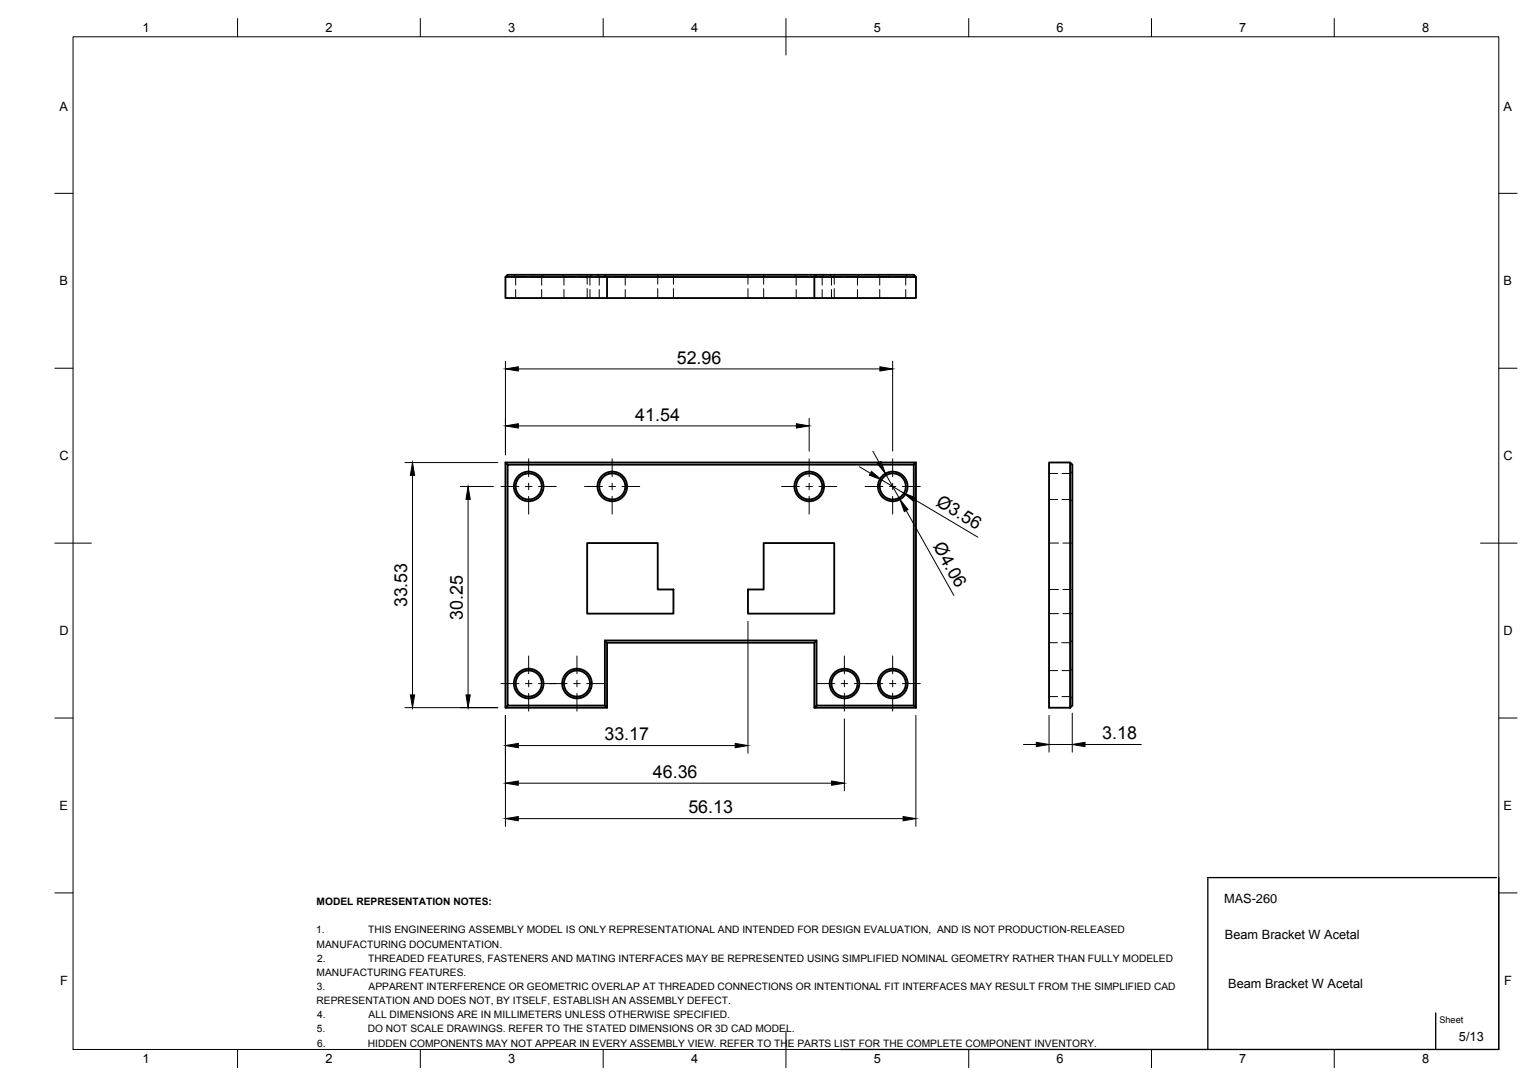
ISO-10303-21;
HEADER;
/* Generated by software containing ST-Developer
 * from STEP Tools, Inc. (www.steptools.com) 
 */

FILE_DESCRIPTION(
/* description */ (''),
/* implementation_level */ '2;1');

FILE_NAME(
/* name */ 'Beam Bracket W Acetal.step',
/* time_stamp */ '2026-10-15T13:29:10-07:00',
/* author */ (''),
/* organization */ (''),
/* preprocessor_version */ 'ST-DEVELOPER v20.2',
/* originating_system */ 'Autodesk Translation Framework v15.15.0.0',
/* authorisation */ '');

FILE_SCHEMA (('AUTOMOTIVE_DESIGN { 1 0 10303 214 3 1 1 }'));
ENDSEC;

DATA;
#10=MECHANICAL_DESIGN_GEOMETRIC_PRESENTATION_REPRESENTATION('',(#940),#83219);
#912=SHAPE_REPRESENTATION_RELATIONSHIP('SRR','None',#83307,#926);
#926=ADVANCED_BREP_SHAPE_REPRESENTATION('',(#954),#83212);
#940=STYLED_ITEM('',(#83386),#954);
#954=MANIFOLD_SOLID_BREP('Body1',#26936);
#1081=FACE_BOUND('',#4704,.T.);
#1082=FACE_BOUND('',#4705,.T.);
#1083=FACE_BOUND('',#4706,.T.);
#1084=FACE_BOUND('',#4707,.T.);
#1085=FACE_BOUND('',#4708,.T.);
#1086=FACE_BOUND('',#4709,.T.);
#1087=FACE_BOUND('',#4710,.T.);
#1088=FACE_BOUND('',#4711,.T.);
#1089=FACE_BOUND('',#4712,.T.);
#1090=FACE_BOUND('',#4713,.T.);
#1091=FACE_BOUND('',#4758,.T.);
#1092=FACE_BOUND('',#4759,.T.);
#1093=FACE_BOUND('',#4760,.T.);
#1094=FACE_BOUND('',#4761,.T.);
#1095=FACE_BOUND('',#4762,.T.);
#1096=FACE_BOUND('',#4763,.T.);
#1097=FACE_BOUND('',#4764,.T.);
#1098=FACE_BOUND('',#4765,.T.);
#1099=FACE_BOUND('',#4766,.T.);
#1100=FACE_BOUND('',#4767,.T.);
#1713=PLANE('',#28339);
#1714=PLANE('',#28377);
#1715=PLANE('',#28378);
#1716=PLANE('',#28379);
#1717=PLANE('',#28380);
#1718=PLANE('',#28381);
#1719=PLANE('',#28382);
#1720=PLANE('',#28383);
#1721=PLANE('',#28384);
#1722=PLANE('',#28385);
#1723=PLANE('',#28386);
#1724=PLANE('',#28387);
#1725=PLANE('',#28388);
#1726=PLANE('',#28389);
#1727=PLANE('',#28390);
#1728=PLANE('',#28391);
#1729=PLANE('',#28392);
#1730=PLANE('',#28393);
#1731=PLANE('',#28394);
#1732=PLANE('',#28395);
#1733=PLANE('',#28396);
#1734=PLANE('',#28397);
#1735=PLANE('',#28398);
#1736=PLANE('',#28399);
#1737=PLANE('',#28400);
#1738=PLANE('',#28401);
#1739=PLANE('',#28402);
#1740=PLANE('',#28403);
#1741=PLANE('',#28404);
#1742=PLANE('',#28405);
#2294=CYLINDRICAL_SURFACE('',#28347,1.778);
#2295=CYLINDRICAL_SURFACE('',#28351,1.778);
#2296=CYLINDRICAL_SURFACE('',#28355,1.778);
#2297=CYLINDRICAL_SURFACE('',#28359,1.778);
#2298=CYLINDRICAL_SURFACE('',#28363,1.778);
#2299=CYLINDRICAL_SURFACE('',#28367,1.778);
#2300=CYLINDRICAL_SURFACE('',#28371,1.778);
#2301=CYLINDRICAL_SURFACE('',#28375,1.778);
#3203=FACE_OUTER_BOUND('',#4702,.T.);
#3204=FACE_OUTER_BOUND('',#4703,.T.);
#3205=FACE_OUTER_BOUND('',#4714,.T.);
#3206=FACE_OUTER_BOUND('',#4715,.T.);
#3207=FACE_OUTER_BOUND('',#4716,.T.);
#3208=FACE_OUTER_BOUND('',#4717,.T.);
#3209=FACE_OUTER_BOUND('',#4718,.T.);
#3210=FACE_OUTER_BOUND('',#4719,.T.);
#3211=FACE_OUTER_BOUND('',#4720,.T.);
#3212=FACE_OUTER_BOUND('',#4721,.T.);
#3213=FACE_OUTER_BOUND('',#4722,.T.);
#3214=FACE_OUTER_BOUND('',#4723,.T.);
#3215=FACE_OUTER_BOUND('',#4724,.T.);
#3216=FACE_OUTER_BOUND('',#4725,.T.);
#3217=FACE_OUTER_BOUND('',#4726,.T.);
#3218=FACE_OUTER_BOUND('',#4727,.T.);
#3219=FACE_OUTER_BOUND('',#4728,.T.);
#3220=FACE_OUTER_BOUND('',#4729,.T.);
#3221=FACE_OUTER_BOUND('',#4730,.T.);
#3222=FACE_OUTER_BOUND('',#4731,.T.);
#3223=FACE_OUTER_BOUND('',#4732,.T.);
#3224=FACE_OUTER_BOUND('',#4733,.T.);
#3225=FACE_OUTER_BOUND('',#4734,.T.);
#3226=FACE_OUTER_BOUND('',#4735,.T.);
#3227=FACE_OUTER_BOUND('',#4736,.T.);
#3228=FACE_OUTER_BOUND('',#4737,.T.);
#3229=FACE_OUTER_BOUND('',#4738,.T.);
#3230=FACE_OUTER_BOUND('',#4739,.T.);
#3231=FACE_OUTER_BOUND('',#4740,.T.);
#3232=FACE_OUTER_BOUND('',#4741,.T.);
#3233=FACE_OUTER_BOUND('',#4742,.T.);
#3234=FACE_OUTER_BOUND('',#4743,.T.);
#3235=FACE_OUTER_BOUND('',#4744,.T.);
#3236=FACE_OUTER_BOUND('',#4745,.T.);
#3237=FACE_OUTER_BOUND('',#4746,.T.);
#3238=FACE_OUTER_BOUND('',#4747,.T.);
#3239=FACE_OUTER_BOUND('',#4748,.T.);
#3240=FACE_OUTER_BOUND('',#4749,.T.);
#3241=FACE_OUTER_BOUND('',#4750,.T.);
#3242=FACE_OUTER_BOUND('',#4751,.T.);
#3243=FACE_OUTER_BOUND('',#4752,.T.);
#3244=FACE_OUTER_BOUND('',#4753,.T.);
#3245=FACE_OUTER_BOUND('',#4754,.T.);
#3246=FACE_OUTER_BOUND('',#4755,.T.);
#3247=FACE_OUTER_BOUND('',#4756,.T.);
#3248=FACE_OUTER_BOUND('',#4757,.T.);
#4702=EDGE_LOOP('',(#22282,#22283,#22284,#22285));
#4703=EDGE_LOOP('',(#22286,#22287,#22288,#22289,#22290,#22291,#22292,#22293));
#4704=EDGE_LOOP('',(#22294));
#4705=EDGE_LOOP('',(#22295));
#4706=EDGE_LOOP('',(#22296));
#4707=EDGE_LOOP('',(#22297));
#4708=EDGE_LOOP('',(#22298,#22299,#22300,#22301,#22302,#22303));
#4709=EDGE_LOOP('',(#22304,#22305,#22306,#22307,#22308,#22309));
#4710=EDGE_LOOP('',(#22310));
#4711=EDGE_LOOP('',(#22311));
#4712=EDGE_LOOP('',(#22312));
#4713=EDGE_LOOP('',(#22313));
#4714=EDGE_LOOP('',(#22314,#22315,#22316,#22317));
#4715=EDGE_LOOP('',(#22318,#22319,#22320,#22321));
#4716=EDGE_LOOP('',(#22322,#22323,#22324,#22325));
#4717=EDGE_LOOP('',(#22326,#22327,#22328,#22329));
#4718=EDGE_LOOP('',(#22330,#22331,#22332,#22333));
#4719=EDGE_LOOP('',(#22334,#22335,#22336,#22337));
#4720=EDGE_LOOP('',(#22338,#22339,#22340,#22341));
#4721=EDGE_LOOP('',(#22342,#22343,#22344,#22345));
#4722=EDGE_LOOP('',(#22346,#22347,#22348,#22349));
#4723=EDGE_LOOP('',(#22350,#22351,#22352,#22353));
#4724=EDGE_LOOP('',(#22354,#22355,#22356,#22357));
#4725=EDGE_LOOP('',(#22358,#22359,#22360,#22361));
#4726=EDGE_LOOP('',(#22362,#22363,#22364,#22365));
#4727=EDGE_LOOP('',(#22366,#22367,#22368,#22369));
#4728=EDGE_LOOP('',(#22370,#22371,#22372,#22373));
#4729=EDGE_LOOP('',(#22374,#22375,#22376,#22377));
#4730=EDGE_LOOP('',(#22378,#22379,#22380,#22381));
#4731=EDGE_LOOP('',(#22382,#22383,#22384,#22385));
#4732=EDGE_LOOP('',(#22386,#22387,#22388,#22389));
#4733=EDGE_LOOP('',(#22390,#22391,#22392,#22393));
#4734=EDGE_LOOP('',(#22394,#22395,#22396,#22397));
#4735=EDGE_LOOP('',(#22398,#22399,#22400,#22401));
#4736=EDGE_LOOP('',(#22402,#22403,#22404,#22405));
#4737=EDGE_LOOP('',(#22406,#22407,#22408,#22409));
#4738=EDGE_LOOP('',(#22410,#22411,#22412,#22413));
#4739=EDGE_LOOP('',(#22414,#22415,#22416,#22417));
#4740=EDGE_LOOP('',(#22418,#22419,#22420,#22421));
#4741=EDGE_LOOP('',(#22422,#22423,#22424,#22425));
#4742=EDGE_LOOP('',(#22426,#22427,#22428,#22429));
#4743=EDGE_LOOP('',(#22430,#22431,#22432,#22433));
#4744=EDGE_LOOP('',(#22434,#22435,#22436,#22437));
#4745=EDGE_LOOP('',(#22438,#22439,#22440,#22441));
#4746=EDGE_LOOP('',(#22442,#22443,#22444,#22445));
#4747=EDGE_LOOP('',(#22446,#22447,#22448,#22449));
#4748=EDGE_LOOP('',(#22450,#22451,#22452,#22453));
#4749=EDGE_LOOP('',(#22454,#22455,#22456,#22457));
#4750=EDGE_LOOP('',(#22458,#22459,#22460,#22461));
#4751=EDGE_LOOP('',(#22462,#22463,#22464,#22465));
#4752=EDGE_LOOP('',(#22466,#22467,#22468,#22469));
#4753=EDGE_LOOP('',(#22470,#22471,#22472,#22473));
#4754=EDGE_LOOP('',(#22474,#22475,#22476,#22477));
#4755=EDGE_LOOP('',(#22478,#22479,#22480,#22481));
#4756=EDGE_LOOP('',(#22482,#22483,#22484,#22485));
#4757=EDGE_LOOP('',(#22486,#22487,#22488,#22489,#22490,#22491,#22492,#22493));
#4758=EDGE_LOOP('',(#22494,#22495,#22496,#22497,#22498,#22499));
#4759=EDGE_LOOP('',(#22500,#22501,#22502,#22503,#22504,#22505));
#4760=EDGE_LOOP('',(#22506));
#4761=EDGE_LOOP('',(#22507));
#4762=EDGE_LOOP('',(#22508));
#4763=EDGE_LOOP('',(#22509));
#4764=EDGE_LOOP('',(#22510));
#4765=EDGE_LOOP('',(#22511));
#4766=EDGE_LOOP('',(#22512));
#4767=EDGE_LOOP('',(#22513));
#6991=LINE('',#52756,#9502);
#6992=LINE('',#52761,#9503);
#6993=LINE('',#52763,#9504);
#6994=LINE('',#52765,#9505);
#6995=LINE('',#52767,#9506);
#6996=LINE('',#52769,#9507);
#6997=LINE('',#52771,#9508);
#6998=LINE('',#52773,#9509);
#6999=LINE('',#52774,#9510);
#7000=LINE('',#52785,#9511);
#7001=LINE('',#52787,#9512);
#7002=LINE('',#52789,#9513);
#7003=LINE('',#52791,#9514);
#7004=LINE('',#52793,#9515);
#7005=LINE('',#52794,#9516);
#7006=LINE('',#52797,#9517);
#7007=LINE('',#52799,#9518);
#7008=LINE('',#52801,#9519);
#7009=LINE('',#52803,#9520);
#7010=LINE('',#52805,#9521);
#7011=LINE('',#52806,#9522);
#7012=LINE('',#52815,#9523);
#7013=LINE('',#52820,#9524);
#7014=LINE('',#52823,#9525);
#7015=LINE('',#52828,#9526);
#7016=LINE('',#52831,#9527);
#7017=LINE('',#52836,#9528);
#7018=LINE('',#52839,#9529);
#7019=LINE('',#52844,#9530);
#7020=LINE('',#52847,#9531);
#7021=LINE('',#52852,#9532);
#7022=LINE('',#52855,#9533);
#7023=LINE('',#52860,#9534);
#7024=LINE('',#52863,#9535);
#7025=LINE('',#52868,#9536);
#7026=LINE('',#52871,#9537);
#7027=LINE('',#52876,#9538);
#7028=LINE('',#52877,#9539);
#7029=LINE('',#52878,#9540);
#7030=LINE('',#52881,#9541);
#7031=LINE('',#52882,#9542);
#7032=LINE('',#52885,#9543);
#7033=LINE('',#52886,#9544);
#7034=LINE('',#52889,#9545);
#7035=LINE('',#52890,#9546);
#7036=LINE('',#52893,#9547);
#7037=LINE('',#52894,#9548);
#7038=LINE('',#52896,#9549);
#7039=LINE('',#52900,#9550);
#7040=LINE('',#52901,#9551);
#7041=LINE('',#52902,#9552);
#7042=LINE('',#52905,#9553);
#7043=LINE('',#52906,#9554);
#7044=LINE('',#52909,#9555);
#7045=LINE('',#52910,#9556);
#7046=LINE('',#52913,#9557);
#7047=LINE('',#52914,#9558);
#7048=LINE('',#52917,#9559);
#7049=LINE('',#52918,#9560);
#7050=LINE('',#52920,#9561);
#7051=LINE('',#52923,#9562);
#7052=LINE('',#52925,#9563);
#7053=LINE('',#52926,#9564);
#7054=LINE('',#52929,#9565);
#7055=LINE('',#52930,#9566);
#7056=LINE('',#52933,#9567);
#7057=LINE('',#52934,#9568);
#7058=LINE('',#52937,#9569);
#7059=LINE('',#52938,#9570);
#7060=LINE('',#52941,#9571);
#7061=LINE('',#52942,#9572);
#7062=LINE('',#52945,#9573);
#7063=LINE('',#52946,#9574);
#7064=LINE('',#52949,#9575);
#7065=LINE('',#52950,#9576);
#7066=LINE('',#52952,#9577);
#7067=LINE('',#52955,#9578);
#7068=LINE('',#52957,#9579);
#7069=LINE('',#52958,#9580);
#7070=LINE('',#52961,#9581);
#7071=LINE('',#52962,#9582);
#7072=LINE('',#52965,#9583);
#7073=LINE('',#52966,#9584);
#7074=LINE('',#52969,#9585);
#7075=LINE('',#52970,#9586);
#7076=LINE('',#52973,#9587);
#7077=LINE('',#52974,#9588);
#7078=LINE('',#52977,#9589);
#7079=LINE('',#52978,#9590);
#7080=LINE('',#52981,#9591);
#7081=LINE('',#52982,#9592);
#7082=LINE('',#52984,#9593);
#9502=VECTOR('',#33449,1.903);
#9503=VECTOR('',#33454,10.);
#9504=VECTOR('',#33455,10.);
#9505=VECTOR('',#33456,10.);
#9506=VECTOR('',#33457,10.);
#9507=VECTOR('',#33458,10.);
#9508=VECTOR('',#33459,10.);
#9509=VECTOR('',#33460,10.);
#9510=VECTOR('',#33461,10.);
#9511=VECTOR('',#33470,10.);
#9512=VECTOR('',#33471,10.);
#9513=VECTOR('',#33472,10.);
#9514=VECTOR('',#33473,10.);
#9515=VECTOR('',#33474,10.);
#9516=VECTOR('',#33475,10.);
#9517=VECTOR('',#33476,10.);
#9518=VECTOR('',#33477,10.);
#9519=VECTOR('',#33478,10.);
#9520=VECTOR('',#33479,10.);
#9521=VECTOR('',#33480,10.);
#9522=VECTOR('',#33481,10.);
#9523=VECTOR('',#33490,1.778);
#9524=VECTOR('',#33497,1.903);
#9525=VECTOR('',#33500,1.778);
#9526=VECTOR('',#33507,1.903);
#9527=VECTOR('',#33510,1.778);
#9528=VECTOR('',#33517,1.903);
#9529=VECTOR('',#33520,1.778);
#9530=VECTOR('',#33527,1.903);
#9531=VECTOR('',#33530,1.778);
#9532=VECTOR('',#33537,1.903);
#9533=VECTOR('',#33540,1.778);
#9534=VECTOR('',#33547,1.903);
#9535=VECTOR('',#33550,1.778);
#9536=VECTOR('',#33557,1.903);
#9537=VECTOR('',#33560,1.778);
#9538=VECTOR('',#33565,10.);
#9539=VECTOR('',#33566,10.);
#9540=VECTOR('',#33567,10.);
#9541=VECTOR('',#33570,10.);
#9542=VECTOR('',#33571,10.);
#9543=VECTOR('',#33574,10.);
#9544=VECTOR('',#33575,10.);
#9545=VECTOR('',#33578,10.);
#9546=VECTOR('',#33579,10.);
#9547=VECTOR('',#33582,10.);
#9548=VECTOR('',#33583,10.);
#9549=VECTOR('',#33586,10.);
#9550=VECTOR('',#33589,10.);
#9551=VECTOR('',#33590,10.);
#9552=VECTOR('',#33591,10.);
#9553=VECTOR('',#33594,10.);
#9554=VECTOR('',#33595,10.);
#9555=VECTOR('',#33598,10.);
#9556=VECTOR('',#33599,10.);
#9557=VECTOR('',#33602,10.);
#9558=VECTOR('',#33603,10.);
#9559=VECTOR('',#33606,10.);
#9560=VECTOR('',#33607,10.);
#9561=VECTOR('',#33610,10.);
#9562=VECTOR('',#33613,10.);
#9563=VECTOR('',#33614,10.);
#9564=VECTOR('',#33615,10.);
#9565=VECTOR('',#33618,10.);
#9566=VECTOR('',#33619,10.);
#9567=VECTOR('',#33622,10.);
#9568=VECTOR('',#33623,10.);
#9569=VECTOR('',#33626,10.);
#9570=VECTOR('',#33627,10.);
#9571=VECTOR('',#33630,10.);
#9572=VECTOR('',#33631,10.);
#9573=VECTOR('',#33634,10.);
#9574=VECTOR('',#33635,10.);
#9575=VECTOR('',#33638,10.);
#9576=VECTOR('',#33639,10.);
#9577=VECTOR('',#33642,10.);
#9578=VECTOR('',#33645,10.);
#9579=VECTOR('',#33646,10.);
#9580=VECTOR('',#33647,10.);
#9581=VECTOR('',#33650,10.);
#9582=VECTOR('',#33651,10.);
#9583=VECTOR('',#33654,10.);
#9584=VECTOR('',#33655,10.);
#9585=VECTOR('',#33658,10.);
#9586=VECTOR('',#33659,10.);
#9587=VECTOR('',#33662,10.);
#9588=VECTOR('',#33663,10.);
#9589=VECTOR('',#33666,10.);
#9590=VECTOR('',#33667,10.);
#9591=VECTOR('',#33670,10.);
#9592=VECTOR('',#33671,10.);
#9593=VECTOR('',#33674,10.);
#10716=CIRCLE('',#28337,1.778);
#10717=CIRCLE('',#28338,2.028);
#10718=CIRCLE('',#28340,2.028);
#10719=CIRCLE('',#28341,2.028);
#10720=CIRCLE('',#28342,2.028);
#10721=CIRCLE('',#28343,2.028);
#10722=CIRCLE('',#28344,2.028);
#10723=CIRCLE('',#28345,2.028);
#10724=CIRCLE('',#28346,2.028);
#10725=CIRCLE('',#28348,1.778);
#10726=CIRCLE('',#28350,1.778);
#10727=CIRCLE('',#28352,1.778);
#10728=CIRCLE('',#28354,1.778);
#10729=CIRCLE('',#28356,1.778);
#10730=CIRCLE('',#28358,1.778);
#10731=CIRCLE('',#28360,1.778);
#10732=CIRCLE('',#28362,1.778);
#10733=CIRCLE('',#28364,1.778);
#10734=CIRCLE('',#28366,1.778);
#10735=CIRCLE('',#28368,1.778);
#10736=CIRCLE('',#28370,1.778);
#10737=CIRCLE('',#28372,1.778);
#10738=CIRCLE('',#28374,1.778);
#10739=CIRCLE('',#28376,1.778);
#12579=VERTEX_POINT('',#52753);
#12580=VERTEX_POINT('',#52755);
#12581=VERTEX_POINT('',#52759);
#12582=VERTEX_POINT('',#52760);
#12583=VERTEX_POINT('',#52762);
#12584=VERTEX_POINT('',#52764);
#12585=VERTEX_POINT('',#52766);
#12586=VERTEX_POINT('',#52768);
#12587=VERTEX_POINT('',#52770);
#12588=VERTEX_POINT('',#52772);
#12589=VERTEX_POINT('',#52775);
#12590=VERTEX_POINT('',#52777);
#12591=VERTEX_POINT('',#52779);
#12592=VERTEX_POINT('',#52781);
#12593=VERTEX_POINT('',#52783);
#12594=VERTEX_POINT('',#52784);
#12595=VERTEX_POINT('',#52786);
#12596=VERTEX_POINT('',#52788);
#12597=VERTEX_POINT('',#52790);
#12598=VERTEX_POINT('',#52792);
#12599=VERTEX_POINT('',#52795);
#12600=VERTEX_POINT('',#52796);
#12601=VERTEX_POINT('',#52798);
#12602=VERTEX_POINT('',#52800);
#12603=VERTEX_POINT('',#52802);
#12604=VERTEX_POINT('',#52804);
#12605=VERTEX_POINT('',#52807);
#12606=VERTEX_POINT('',#52809);
#12607=VERTEX_POINT('',#52811);
#12608=VERTEX_POINT('',#52814);
#12609=VERTEX_POINT('',#52818);
#12610=VERTEX_POINT('',#52822);
#12611=VERTEX_POINT('',#52826);
#12612=VERTEX_POINT('',#52830);
#12613=VERTEX_POINT('',#52834);
#12614=VERTEX_POINT('',#52838);
#12615=VERTEX_POINT('',#52842);
#12616=VERTEX_POINT('',#52846);
#12617=VERTEX_POINT('',#52850);
#12618=VERTEX_POINT('',#52854);
#12619=VERTEX_POINT('',#52858);
#12620=VERTEX_POINT('',#52862);
#12621=VERTEX_POINT('',#52866);
#12622=VERTEX_POINT('',#52870);
#12623=VERTEX_POINT('',#52874);
#12624=VERTEX_POINT('',#52875);
#12625=VERTEX_POINT('',#52880);
#12626=VERTEX_POINT('',#52884);
#12627=VERTEX_POINT('',#52888);
#12628=VERTEX_POINT('',#52892);
#12629=VERTEX_POINT('',#52898);
#12630=VERTEX_POINT('',#52899);
#12631=VERTEX_POINT('',#52904);
#12632=VERTEX_POINT('',#52908);
#12633=VERTEX_POINT('',#52912);
#12634=VERTEX_POINT('',#52916);
#12635=VERTEX_POINT('',#52922);
#12636=VERTEX_POINT('',#52924);
#12637=VERTEX_POINT('',#52928);
#12638=VERTEX_POINT('',#52932);
#12639=VERTEX_POINT('',#52936);
#12640=VERTEX_POINT('',#52940);
#12641=VERTEX_POINT('',#52944);
#12642=VERTEX_POINT('',#52948);
#12643=VERTEX_POINT('',#52954);
#12644=VERTEX_POINT('',#52956);
#12645=VERTEX_POINT('',#52960);
#12646=VERTEX_POINT('',#52964);
#12647=VERTEX_POINT('',#52968);
#12648=VERTEX_POINT('',#52972);
#12649=VERTEX_POINT('',#52976);
#12650=VERTEX_POINT('',#52980);
#16002=EDGE_CURVE('',#12579,#12579,#10716,.T.);
#16003=EDGE_CURVE('',#12579,#12580,#6991,.T.);
#16004=EDGE_CURVE('',#12580,#12580,#10717,.T.);
#16005=EDGE_CURVE('',#12581,#12582,#6992,.T.);
#16006=EDGE_CURVE('',#12583,#12581,#6993,.T.);
#16007=EDGE_CURVE('',#12584,#12583,#6994,.T.);
#16008=EDGE_CURVE('',#12585,#12584,#6995,.T.);
#16009=EDGE_CURVE('',#12586,#12585,#6996,.T.);
#16010=EDGE_CURVE('',#12587,#12586,#6997,.T.);
#16011=EDGE_CURVE('',#12588,#12587,#6998,.T.);
#16012=EDGE_CURVE('',#12582,#12588,#6999,.T.);
#16013=EDGE_CURVE('',#12589,#12589,#10718,.T.);
#16014=EDGE_CURVE('',#12590,#12590,#10719,.T.);
#16015=EDGE_CURVE('',#12591,#12591,#10720,.T.);
#16016=EDGE_CURVE('',#12592,#12592,#10721,.T.);
#16017=EDGE_CURVE('',#12593,#12594,#7000,.T.);
#16018=EDGE_CURVE('',#12594,#12595,#7001,.T.);
#16019=EDGE_CURVE('',#12595,#12596,#7002,.T.);
#16020=EDGE_CURVE('',#12596,#12597,#7003,.T.);
#16021=EDGE_CURVE('',#12597,#12598,#7004,.T.);
#16022=EDGE_CURVE('',#12598,#12593,#7005,.T.);
#16023=EDGE_CURVE('',#12599,#12600,#7006,.T.);
#16024=EDGE_CURVE('',#12600,#12601,#7007,.T.);
#16025=EDGE_CURVE('',#12601,#12602,#7008,.T.);
#16026=EDGE_CURVE('',#12602,#12603,#7009,.T.);
#16027=EDGE_CURVE('',#12603,#12604,#7010,.T.);
#16028=EDGE_CURVE('',#12604,#12599,#7011,.T.);
#16029=EDGE_CURVE('',#12605,#12605,#10722,.T.);
#16030=EDGE_CURVE('',#12606,#12606,#10723,.T.);
#16031=EDGE_CURVE('',#12607,#12607,#10724,.T.);
#16032=EDGE_CURVE('',#12579,#12608,#7012,.T.);
#16033=EDGE_CURVE('',#12608,#12608,#10725,.T.);
#16034=EDGE_CURVE('',#12609,#12609,#10726,.T.);
#16035=EDGE_CURVE('',#12609,#12589,#7013,.T.);
#16036=EDGE_CURVE('',#12609,#12610,#7014,.T.);
#16037=EDGE_CURVE('',#12610,#12610,#10727,.T.);
#16038=EDGE_CURVE('',#12611,#12611,#10728,.T.);
#16039=EDGE_CURVE('',#12611,#12607,#7015,.T.);
#16040=EDGE_CURVE('',#12611,#12612,#7016,.T.);
#16041=EDGE_CURVE('',#12612,#12612,#10729,.T.);
#16042=EDGE_CURVE('',#12613,#12613,#10730,.T.);
#16043=EDGE_CURVE('',#12613,#12590,#7017,.T.);
#16044=EDGE_CURVE('',#12613,#12614,#7018,.T.);
#16045=EDGE_CURVE('',#12614,#12614,#10731,.T.);
#16046=EDGE_CURVE('',#12615,#12615,#10732,.T.);
#16047=EDGE_CURVE('',#12615,#12606,#7019,.T.);
#16048=EDGE_CURVE('',#12615,#12616,#7020,.T.);
#16049=EDGE_CURVE('',#12616,#12616,#10733,.T.);
#16050=EDGE_CURVE('',#12617,#12617,#10734,.T.);
#16051=EDGE_CURVE('',#12617,#12591,#7021,.T.);
#16052=EDGE_CURVE('',#12617,#12618,#7022,.T.);
#16053=EDGE_CURVE('',#12618,#12618,#10735,.T.);
#16054=EDGE_CURVE('',#12619,#12619,#10736,.T.);
#16055=EDGE_CURVE('',#12619,#12605,#7023,.T.);
#16056=EDGE_CURVE('',#12619,#12620,#7024,.T.);
#16057=EDGE_CURVE('',#12620,#12620,#10737,.T.);
#16058=EDGE_CURVE('',#12621,#12621,#10738,.T.);
#16059=EDGE_CURVE('',#12621,#12592,#7025,.T.);
#16060=EDGE_CURVE('',#12621,#12622,#7026,.T.);
#16061=EDGE_CURVE('',#12622,#12622,#10739,.T.);
#16062=EDGE_CURVE('',#12623,#12624,#7027,.T.);
#16063=EDGE_CURVE('',#12623,#12600,#7028,.T.);
#16064=EDGE_CURVE('',#12624,#12599,#7029,.T.);
#16065=EDGE_CURVE('',#12625,#12623,#7030,.T.);
#16066=EDGE_CURVE('',#12625,#12601,#7031,.T.);
#16067=EDGE_CURVE('',#12626,#12625,#7032,.T.);
#16068=EDGE_CURVE('',#12626,#12602,#7033,.T.);
#16069=EDGE_CURVE('',#12627,#12626,#7034,.T.);
#16070=EDGE_CURVE('',#12627,#12603,#7035,.T.);
#16071=EDGE_CURVE('',#12628,#12627,#7036,.T.);
#16072=EDGE_CURVE('',#12628,#12604,#7037,.T.);
#16073=EDGE_CURVE('',#12624,#12628,#7038,.T.);
#16074=EDGE_CURVE('',#12629,#12630,#7039,.T.);
#16075=EDGE_CURVE('',#12629,#12594,#7040,.T.);
#16076=EDGE_CURVE('',#12630,#12593,#7041,.T.);
#16077=EDGE_CURVE('',#12631,#12629,#7042,.T.);
#16078=EDGE_CURVE('',#12631,#12595,#7043,.T.);
#16079=EDGE_CURVE('',#12632,#12631,#7044,.T.);
#16080=EDGE_CURVE('',#12632,#12596,#7045,.T.);
#16081=EDGE_CURVE('',#12633,#12632,#7046,.T.);
#16082=EDGE_CURVE('',#12633,#12597,#7047,.T.);
#16083=EDGE_CURVE('',#12634,#12633,#7048,.T.);
#16084=EDGE_CURVE('',#12634,#12598,#7049,.T.);
#16085=EDGE_CURVE('',#12630,#12634,#7050,.T.);
#16086=EDGE_CURVE('',#12582,#12635,#7051,.T.);
#16087=EDGE_CURVE('',#12635,#12636,#7052,.T.);
#16088=EDGE_CURVE('',#12581,#12636,#7053,.T.);
#16089=EDGE_CURVE('',#12588,#12637,#7054,.T.);
#16090=EDGE_CURVE('',#12637,#12635,#7055,.T.);
#16091=EDGE_CURVE('',#12587,#12638,#7056,.T.);
#16092=EDGE_CURVE('',#12638,#12637,#7057,.T.);
#16093=EDGE_CURVE('',#12586,#12639,#7058,.T.);
#16094=EDGE_CURVE('',#12639,#12638,#7059,.T.);
#16095=EDGE_CURVE('',#12585,#12640,#7060,.T.);
#16096=EDGE_CURVE('',#12640,#12639,#7061,.T.);
#16097=EDGE_CURVE('',#12641,#12640,#7062,.T.);
#16098=EDGE_CURVE('',#12584,#12641,#7063,.T.);
#16099=EDGE_CURVE('',#12642,#12641,#7064,.T.);
#16100=EDGE_CURVE('',#12583,#12642,#7065,.T.);
#16101=EDGE_CURVE('',#12636,#12642,#7066,.T.);
#16102=EDGE_CURVE('',#12643,#12641,#7067,.T.);
#16103=EDGE_CURVE('',#12644,#12643,#7068,.T.);
#16104=EDGE_CURVE('',#12644,#12640,#7069,.T.);
#16105=EDGE_CURVE('',#12645,#12642,#7070,.T.);
#16106=EDGE_CURVE('',#12643,#12645,#7071,.T.);
#16107=EDGE_CURVE('',#12646,#12636,#7072,.T.);
#16108=EDGE_CURVE('',#12645,#12646,#7073,.T.);
#16109=EDGE_CURVE('',#12647,#12635,#7074,.T.);
#16110=EDGE_CURVE('',#12646,#12647,#7075,.T.);
#16111=EDGE_CURVE('',#12648,#12644,#7076,.T.);
#16112=EDGE_CURVE('',#12648,#12639,#7077,.T.);
#16113=EDGE_CURVE('',#12649,#12637,#7078,.T.);
#16114=EDGE_CURVE('',#12647,#12649,#7079,.T.);
#16115=EDGE_CURVE('',#12650,#12638,#7080,.T.);
#16116=EDGE_CURVE('',#12649,#12650,#7081,.T.);
#16117=EDGE_CURVE('',#12650,#12648,#7082,.T.);
#22282=ORIENTED_EDGE('',*,*,#16002,.T.);
#22283=ORIENTED_EDGE('',*,*,#16003,.T.);
#22284=ORIENTED_EDGE('',*,*,#16004,.T.);
#22285=ORIENTED_EDGE('',*,*,#16003,.F.);
#22286=ORIENTED_EDGE('',*,*,#16005,.F.);
#22287=ORIENTED_EDGE('',*,*,#16006,.F.);
#22288=ORIENTED_EDGE('',*,*,#16007,.F.);
#22289=ORIENTED_EDGE('',*,*,#16008,.F.);
#22290=ORIENTED_EDGE('',*,*,#16009,.F.);
#22291=ORIENTED_EDGE('',*,*,#16010,.F.);
#22292=ORIENTED_EDGE('',*,*,#16011,.F.);
#22293=ORIENTED_EDGE('',*,*,#16012,.F.);
#22294=ORIENTED_EDGE('',*,*,#16013,.F.);
#22295=ORIENTED_EDGE('',*,*,#16014,.F.);
#22296=ORIENTED_EDGE('',*,*,#16015,.F.);
#22297=ORIENTED_EDGE('',*,*,#16016,.F.);
#22298=ORIENTED_EDGE('',*,*,#16017,.T.);
#22299=ORIENTED_EDGE('',*,*,#16018,.T.);
#22300=ORIENTED_EDGE('',*,*,#16019,.T.);
#22301=ORIENTED_EDGE('',*,*,#16020,.T.);
#22302=ORIENTED_EDGE('',*,*,#16021,.T.);
#22303=ORIENTED_EDGE('',*,*,#16022,.T.);
#22304=ORIENTED_EDGE('',*,*,#16023,.T.);
#22305=ORIENTED_EDGE('',*,*,#16024,.T.);
#22306=ORIENTED_EDGE('',*,*,#16025,.T.);
#22307=ORIENTED_EDGE('',*,*,#16026,.T.);
#22308=ORIENTED_EDGE('',*,*,#16027,.T.);
#22309=ORIENTED_EDGE('',*,*,#16028,.T.);
#22310=ORIENTED_EDGE('',*,*,#16029,.F.);
#22311=ORIENTED_EDGE('',*,*,#16030,.F.);
#22312=ORIENTED_EDGE('',*,*,#16031,.F.);
#22313=ORIENTED_EDGE('',*,*,#16004,.F.);
#22314=ORIENTED_EDGE('',*,*,#16002,.F.);
#22315=ORIENTED_EDGE('',*,*,#16032,.T.);
#22316=ORIENTED_EDGE('',*,*,#16033,.F.);
#22317=ORIENTED_EDGE('',*,*,#16032,.F.);
#22318=ORIENTED_EDGE('',*,*,#16034,.T.);
#22319=ORIENTED_EDGE('',*,*,#16035,.T.);
#22320=ORIENTED_EDGE('',*,*,#16013,.T.);
#22321=ORIENTED_EDGE('',*,*,#16035,.F.);
#22322=ORIENTED_EDGE('',*,*,#16034,.F.);
#22323=ORIENTED_EDGE('',*,*,#16036,.T.);
#22324=ORIENTED_EDGE('',*,*,#16037,.F.);
#22325=ORIENTED_EDGE('',*,*,#16036,.F.);
#22326=ORIENTED_EDGE('',*,*,#16038,.T.);
#22327=ORIENTED_EDGE('',*,*,#16039,.T.);
#22328=ORIENTED_EDGE('',*,*,#16031,.T.);
#22329=ORIENTED_EDGE('',*,*,#16039,.F.);
#22330=ORIENTED_EDGE('',*,*,#16038,.F.);
#22331=ORIENTED_EDGE('',*,*,#16040,.T.);
#22332=ORIENTED_EDGE('',*,*,#16041,.F.);
#22333=ORIENTED_EDGE('',*,*,#16040,.F.);
#22334=ORIENTED_EDGE('',*,*,#16042,.T.);
#22335=ORIENTED_EDGE('',*,*,#16043,.T.);
#22336=ORIENTED_EDGE('',*,*,#16014,.T.);
#22337=ORIENTED_EDGE('',*,*,#16043,.F.);
#22338=ORIENTED_EDGE('',*,*,#16042,.F.);
#22339=ORIENTED_EDGE('',*,*,#16044,.T.);
#22340=ORIENTED_EDGE('',*,*,#16045,.F.);
#22341=ORIENTED_EDGE('',*,*,#16044,.F.);
#22342=ORIENTED_EDGE('',*,*,#16046,.T.);
#22343=ORIENTED_EDGE('',*,*,#16047,.T.);
#22344=ORIENTED_EDGE('',*,*,#16030,.T.);
#22345=ORIENTED_EDGE('',*,*,#16047,.F.);
#22346=ORIENTED_EDGE('',*,*,#16046,.F.);
#22347=ORIENTED_EDGE('',*,*,#16048,.T.);
#22348=ORIENTED_EDGE('',*,*,#16049,.F.);
#22349=ORIENTED_EDGE('',*,*,#16048,.F.);
#22350=ORIENTED_EDGE('',*,*,#16050,.T.);
#22351=ORIENTED_EDGE('',*,*,#16051,.T.);
#22352=ORIENTED_EDGE('',*,*,#16015,.T.);
#22353=ORIENTED_EDGE('',*,*,#16051,.F.);
#22354=ORIENTED_EDGE('',*,*,#16050,.F.);
#22355=ORIENTED_EDGE('',*,*,#16052,.T.);
#22356=ORIENTED_EDGE('',*,*,#16053,.F.);
#22357=ORIENTED_EDGE('',*,*,#16052,.F.);
#22358=ORIENTED_EDGE('',*,*,#16054,.T.);
#22359=ORIENTED_EDGE('',*,*,#16055,.T.);
#22360=ORIENTED_EDGE('',*,*,#16029,.T.);
#22361=ORIENTED_EDGE('',*,*,#16055,.F.);
#22362=ORIENTED_EDGE('',*,*,#16054,.F.);
#22363=ORIENTED_EDGE('',*,*,#16056,.T.);
#22364=ORIENTED_EDGE('',*,*,#16057,.F.);
#22365=ORIENTED_EDGE('',*,*,#16056,.F.);
#22366=ORIENTED_EDGE('',*,*,#16058,.T.);
#22367=ORIENTED_EDGE('',*,*,#16059,.T.);
#22368=ORIENTED_EDGE('',*,*,#16016,.T.);
#22369=ORIENTED_EDGE('',*,*,#16059,.F.);
#22370=ORIENTED_EDGE('',*,*,#16058,.F.);
#22371=ORIENTED_EDGE('',*,*,#16060,.T.);
#22372=ORIENTED_EDGE('',*,*,#16061,.F.);
#22373=ORIENTED_EDGE('',*,*,#16060,.F.);
#22374=ORIENTED_EDGE('',*,*,#16062,.F.);
#22375=ORIENTED_EDGE('',*,*,#16063,.T.);
#22376=ORIENTED_EDGE('',*,*,#16023,.F.);
#22377=ORIENTED_EDGE('',*,*,#16064,.F.);
#22378=ORIENTED_EDGE('',*,*,#16065,.F.);
#22379=ORIENTED_EDGE('',*,*,#16066,.T.);
#22380=ORIENTED_EDGE('',*,*,#16024,.F.);
#22381=ORIENTED_EDGE('',*,*,#16063,.F.);
#22382=ORIENTED_EDGE('',*,*,#16067,.F.);
#22383=ORIENTED_EDGE('',*,*,#16068,.T.);
#22384=ORIENTED_EDGE('',*,*,#16025,.F.);
#22385=ORIENTED_EDGE('',*,*,#16066,.F.);
#22386=ORIENTED_EDGE('',*,*,#16069,.F.);
#22387=ORIENTED_EDGE('',*,*,#16070,.T.);
#22388=ORIENTED_EDGE('',*,*,#16026,.F.);
#22389=ORIENTED_EDGE('',*,*,#16068,.F.);
#22390=ORIENTED_EDGE('',*,*,#16071,.F.);
#22391=ORIENTED_EDGE('',*,*,#16072,.T.);
#22392=ORIENTED_EDGE('',*,*,#16027,.F.);
#22393=ORIENTED_EDGE('',*,*,#16070,.F.);
#22394=ORIENTED_EDGE('',*,*,#16073,.F.);
#22395=ORIENTED_EDGE('',*,*,#16064,.T.);
#22396=ORIENTED_EDGE('',*,*,#16028,.F.);
#22397=ORIENTED_EDGE('',*,*,#16072,.F.);
#22398=ORIENTED_EDGE('',*,*,#16074,.F.);
#22399=ORIENTED_EDGE('',*,*,#16075,.T.);
#22400=ORIENTED_EDGE('',*,*,#16017,.F.);
#22401=ORIENTED_EDGE('',*,*,#16076,.F.);
#22402=ORIENTED_EDGE('',*,*,#16077,.F.);
#22403=ORIENTED_EDGE('',*,*,#16078,.T.);
#22404=ORIENTED_EDGE('',*,*,#16018,.F.);
#22405=ORIENTED_EDGE('',*,*,#16075,.F.);
#22406=ORIENTED_EDGE('',*,*,#16079,.F.);
#22407=ORIENTED_EDGE('',*,*,#16080,.T.);
#22408=ORIENTED_EDGE('',*,*,#16019,.F.);
#22409=ORIENTED_EDGE('',*,*,#16078,.F.);
#22410=ORIENTED_EDGE('',*,*,#16081,.F.);
#22411=ORIENTED_EDGE('',*,*,#16082,.T.);
#22412=ORIENTED_EDGE('',*,*,#16020,.F.);
#22413=ORIENTED_EDGE('',*,*,#16080,.F.);
#22414=ORIENTED_EDGE('',*,*,#16083,.F.);
#22415=ORIENTED_EDGE('',*,*,#16084,.T.);
#22416=ORIENTED_EDGE('',*,*,#16021,.F.);
#22417=ORIENTED_EDGE('',*,*,#16082,.F.);
#22418=ORIENTED_EDGE('',*,*,#16085,.F.);
#22419=ORIENTED_EDGE('',*,*,#16076,.T.);
#22420=ORIENTED_EDGE('',*,*,#16022,.F.);
#22421=ORIENTED_EDGE('',*,*,#16084,.F.);
#22422=ORIENTED_EDGE('',*,*,#16005,.T.);
#22423=ORIENTED_EDGE('',*,*,#16086,.T.);
#22424=ORIENTED_EDGE('',*,*,#16087,.T.);
#22425=ORIENTED_EDGE('',*,*,#16088,.F.);
#22426=ORIENTED_EDGE('',*,*,#16012,.T.);
#22427=ORIENTED_EDGE('',*,*,#16089,.T.);
#22428=ORIENTED_EDGE('',*,*,#16090,.T.);
#22429=ORIENTED_EDGE('',*,*,#16086,.F.);
#22430=ORIENTED_EDGE('',*,*,#16011,.T.);
#22431=ORIENTED_EDGE('',*,*,#16091,.T.);
#22432=ORIENTED_EDGE('',*,*,#16092,.T.);
#22433=ORIENTED_EDGE('',*,*,#16089,.F.);
#22434=ORIENTED_EDGE('',*,*,#16010,.T.);
#22435=ORIENTED_EDGE('',*,*,#16093,.T.);
#22436=ORIENTED_EDGE('',*,*,#16094,.T.);
#22437=ORIENTED_EDGE('',*,*,#16091,.F.);
#22438=ORIENTED_EDGE('',*,*,#16009,.T.);
#22439=ORIENTED_EDGE('',*,*,#16095,.T.);
#22440=ORIENTED_EDGE('',*,*,#16096,.T.);
#22441=ORIENTED_EDGE('',*,*,#16093,.F.);
#22442=ORIENTED_EDGE('',*,*,#16097,.T.);
#22443=ORIENTED_EDGE('',*,*,#16095,.F.);
#22444=ORIENTED_EDGE('',*,*,#16008,.T.);
#22445=ORIENTED_EDGE('',*,*,#16098,.T.);
#22446=ORIENTED_EDGE('',*,*,#16099,.T.);
#22447=ORIENTED_EDGE('',*,*,#16098,.F.);
#22448=ORIENTED_EDGE('',*,*,#16007,.T.);
#22449=ORIENTED_EDGE('',*,*,#16100,.T.);
#22450=ORIENTED_EDGE('',*,*,#16101,.T.);
#22451=ORIENTED_EDGE('',*,*,#16100,.F.);
#22452=ORIENTED_EDGE('',*,*,#16006,.T.);
#22453=ORIENTED_EDGE('',*,*,#16088,.T.);
#22454=ORIENTED_EDGE('',*,*,#16097,.F.);
#22455=ORIENTED_EDGE('',*,*,#16102,.F.);
#22456=ORIENTED_EDGE('',*,*,#16103,.F.);
#22457=ORIENTED_EDGE('',*,*,#16104,.T.);
#22458=ORIENTED_EDGE('',*,*,#16099,.F.);
#22459=ORIENTED_EDGE('',*,*,#16105,.F.);
#22460=ORIENTED_EDGE('',*,*,#16106,.F.);
#22461=ORIENTED_EDGE('',*,*,#16102,.T.);
#22462=ORIENTED_EDGE('',*,*,#16101,.F.);
#22463=ORIENTED_EDGE('',*,*,#16107,.F.);
#22464=ORIENTED_EDGE('',*,*,#16108,.F.);
#22465=ORIENTED_EDGE('',*,*,#16105,.T.);
#22466=ORIENTED_EDGE('',*,*,#16087,.F.);
#22467=ORIENTED_EDGE('',*,*,#16109,.F.);
#22468=ORIENTED_EDGE('',*,*,#16110,.F.);
#22469=ORIENTED_EDGE('',*,*,#16107,.T.);
#22470=ORIENTED_EDGE('',*,*,#16096,.F.);
#22471=ORIENTED_EDGE('',*,*,#16104,.F.);
#22472=ORIENTED_EDGE('',*,*,#16111,.F.);
#22473=ORIENTED_EDGE('',*,*,#16112,.T.);
#22474=ORIENTED_EDGE('',*,*,#16090,.F.);
#22475=ORIENTED_EDGE('',*,*,#16113,.F.);
#22476=ORIENTED_EDGE('',*,*,#16114,.F.);
#22477=ORIENTED_EDGE('',*,*,#16109,.T.);
#22478=ORIENTED_EDGE('',*,*,#16092,.F.);
#22479=ORIENTED_EDGE('',*,*,#16115,.F.);
#22480=ORIENTED_EDGE('',*,*,#16116,.F.);
#22481=ORIENTED_EDGE('',*,*,#16113,.T.);
#22482=ORIENTED_EDGE('',*,*,#16094,.F.);
#22483=ORIENTED_EDGE('',*,*,#16112,.F.);
#22484=ORIENTED_EDGE('',*,*,#16117,.F.);
#22485=ORIENTED_EDGE('',*,*,#16115,.T.);
#22486=ORIENTED_EDGE('',*,*,#16117,.T.);
#22487=ORIENTED_EDGE('',*,*,#16111,.T.);
#22488=ORIENTED_EDGE('',*,*,#16103,.T.);
#22489=ORIENTED_EDGE('',*,*,#16106,.T.);
#22490=ORIENTED_EDGE('',*,*,#16108,.T.);
#22491=ORIENTED_EDGE('',*,*,#16110,.T.);
#22492=ORIENTED_EDGE('',*,*,#16114,.T.);
#22493=ORIENTED_EDGE('',*,*,#16116,.T.);
#22494=ORIENTED_EDGE('',*,*,#16074,.T.);
#22495=ORIENTED_EDGE('',*,*,#16085,.T.);
#22496=ORIENTED_EDGE('',*,*,#16083,.T.);
#22497=ORIENTED_EDGE('',*,*,#16081,.T.);
#22498=ORIENTED_EDGE('',*,*,#16079,.T.);
#22499=ORIENTED_EDGE('',*,*,#16077,.T.);
#22500=ORIENTED_EDGE('',*,*,#16062,.T.);
#22501=ORIENTED_EDGE('',*,*,#16073,.T.);
#22502=ORIENTED_EDGE('',*,*,#16071,.T.);
#22503=ORIENTED_EDGE('',*,*,#16069,.T.);
#22504=ORIENTED_EDGE('',*,*,#16067,.T.);
#22505=ORIENTED_EDGE('',*,*,#16065,.T.);
#22506=ORIENTED_EDGE('',*,*,#16033,.T.);
#22507=ORIENTED_EDGE('',*,*,#16037,.T.);
#22508=ORIENTED_EDGE('',*,*,#16041,.T.);
#22509=ORIENTED_EDGE('',*,*,#16045,.T.);
#22510=ORIENTED_EDGE('',*,*,#16049,.T.);
#22511=ORIENTED_EDGE('',*,*,#16053,.T.);
#22512=ORIENTED_EDGE('',*,*,#16057,.T.);
#22513=ORIENTED_EDGE('',*,*,#16061,.T.);
#25518=CONICAL_SURFACE('',#28336,1.903,0.785398163397448);
#25519=CONICAL_SURFACE('',#28349,1.903,0.785398163397448);
#25520=CONICAL_SURFACE('',#28353,1.903,0.785398163397448);
#25521=CONICAL_SURFACE('',#28357,1.903,0.785398163397448);
#25522=CONICAL_SURFACE('',#28361,1.903,0.785398163397448);
#25523=CONICAL_SURFACE('',#28365,1.903,0.785398163397448);
#25524=CONICAL_SURFACE('',#28369,1.903,0.785398163397448);
#25525=CONICAL_SURFACE('',#28373,1.903,0.785398163397448);
#26396=ADVANCED_FACE('',(#3203),#25518,.F.);
#26397=ADVANCED_FACE('',(#3204,#1081,#1082,#1083,#1084,#1085,#1086,#1087,
#1088,#1089,#1090),#1713,.T.);
#26398=ADVANCED_FACE('',(#3205),#2294,.F.);
#26399=ADVANCED_FACE('',(#3206),#25519,.F.);
#26400=ADVANCED_FACE('',(#3207),#2295,.F.);
#26401=ADVANCED_FACE('',(#3208),#25520,.F.);
#26402=ADVANCED_FACE('',(#3209),#2296,.F.);
#26403=ADVANCED_FACE('',(#3210),#25521,.F.);
#26404=ADVANCED_FACE('',(#3211),#2297,.F.);
#26405=ADVANCED_FACE('',(#3212),#25522,.F.);
#26406=ADVANCED_FACE('',(#3213),#2298,.F.);
#26407=ADVANCED_FACE('',(#3214),#25523,.F.);
#26408=ADVANCED_FACE('',(#3215),#2299,.F.);
#26409=ADVANCED_FACE('',(#3216),#25524,.F.);
#26410=ADVANCED_FACE('',(#3217),#2300,.F.);
#26411=ADVANCED_FACE('',(#3218),#25525,.F.);
#26412=ADVANCED_FACE('',(#3219),#2301,.F.);
#26413=ADVANCED_FACE('',(#3220),#1714,.F.);
#26414=ADVANCED_FACE('',(#3221),#1715,.F.);
#26415=ADVANCED_FACE('',(#3222),#1716,.F.);
#26416=ADVANCED_FACE('',(#3223),#1717,.F.);
#26417=ADVANCED_FACE('',(#3224),#1718,.F.);
#26418=ADVANCED_FACE('',(#3225),#1719,.F.);
#26419=ADVANCED_FACE('',(#3226),#1720,.F.);
#26420=ADVANCED_FACE('',(#3227),#1721,.F.);
#26421=ADVANCED_FACE('',(#3228),#1722,.F.);
#26422=ADVANCED_FACE('',(#3229),#1723,.F.);
#26423=ADVANCED_FACE('',(#3230),#1724,.F.);
#26424=ADVANCED_FACE('',(#3231),#1725,.F.);
#26425=ADVANCED_FACE('',(#3232),#1726,.T.);
#26426=ADVANCED_FACE('',(#3233),#1727,.T.);
#26427=ADVANCED_FACE('',(#3234),#1728,.T.);
#26428=ADVANCED_FACE('',(#3235),#1729,.T.);
#26429=ADVANCED_FACE('',(#3236),#1730,.T.);
#26430=ADVANCED_FACE('',(#3237),#1731,.T.);
#26431=ADVANCED_FACE('',(#3238),#1732,.T.);
#26432=ADVANCED_FACE('',(#3239),#1733,.T.);
#26433=ADVANCED_FACE('',(#3240),#1734,.T.);
#26434=ADVANCED_FACE('',(#3241),#1735,.T.);
#26435=ADVANCED_FACE('',(#3242),#1736,.T.);
#26436=ADVANCED_FACE('',(#3243),#1737,.T.);
#26437=ADVANCED_FACE('',(#3244),#1738,.T.);
#26438=ADVANCED_FACE('',(#3245),#1739,.T.);
#26439=ADVANCED_FACE('',(#3246),#1740,.T.);
#26440=ADVANCED_FACE('',(#3247),#1741,.T.);
#26441=ADVANCED_FACE('',(#3248,#1091,#1092,#1093,#1094,#1095,#1096,#1097,
#1098,#1099,#1100),#1742,.F.);
#26936=CLOSED_SHELL('',(#26396,#26397,#26398,#26399,#26400,#26401,#26402,
#26403,#26404,#26405,#26406,#26407,#26408,#26409,#26410,#26411,#26412,#26413,
#26414,#26415,#26416,#26417,#26418,#26419,#26420,#26421,#26422,#26423,#26424,
#26425,#26426,#26427,#26428,#26429,#26430,#26431,#26432,#26433,#26434,#26435,
#26436,#26437,#26438,#26439,#26440,#26441));
#28335=AXIS2_PLACEMENT_3D('',#52751,#33443,#33444);
#28336=AXIS2_PLACEMENT_3D('',#52752,#33445,#33446);
#28337=AXIS2_PLACEMENT_3D('',#52754,#33447,#33448);
#28338=AXIS2_PLACEMENT_3D('',#52757,#33450,#33451);
#28339=AXIS2_PLACEMENT_3D('',#52758,#33452,#33453);
#28340=AXIS2_PLACEMENT_3D('',#52776,#33462,#33463);
#28341=AXIS2_PLACEMENT_3D('',#52778,#33464,#33465);
#28342=AXIS2_PLACEMENT_3D('',#52780,#33466,#33467);
#28343=AXIS2_PLACEMENT_3D('',#52782,#33468,#33469);
#28344=AXIS2_PLACEMENT_3D('',#52808,#33482,#33483);
#28345=AXIS2_PLACEMENT_3D('',#52810,#33484,#33485);
#28346=AXIS2_PLACEMENT_3D('',#52812,#33486,#33487);
#28347=AXIS2_PLACEMENT_3D('',#52813,#33488,#33489);
#28348=AXIS2_PLACEMENT_3D('',#52816,#33491,#33492);
#28349=AXIS2_PLACEMENT_3D('',#52817,#33493,#33494);
#28350=AXIS2_PLACEMENT_3D('',#52819,#33495,#33496);
#28351=AXIS2_PLACEMENT_3D('',#52821,#33498,#33499);
#28352=AXIS2_PLACEMENT_3D('',#52824,#33501,#33502);
#28353=AXIS2_PLACEMENT_3D('',#52825,#33503,#33504);
#28354=AXIS2_PLACEMENT_3D('',#52827,#33505,#33506);
#28355=AXIS2_PLACEMENT_3D('',#52829,#33508,#33509);
#28356=AXIS2_PLACEMENT_3D('',#52832,#33511,#33512);
#28357=AXIS2_PLACEMENT_3D('',#52833,#33513,#33514);
#28358=AXIS2_PLACEMENT_3D('',#52835,#33515,#33516);
#28359=AXIS2_PLACEMENT_3D('',#52837,#33518,#33519);
#28360=AXIS2_PLACEMENT_3D('',#52840,#33521,#33522);
#28361=AXIS2_PLACEMENT_3D('',#52841,#33523,#33524);
#28362=AXIS2_PLACEMENT_3D('',#52843,#33525,#33526);
#28363=AXIS2_PLACEMENT_3D('',#52845,#33528,#33529);
#28364=AXIS2_PLACEMENT_3D('',#52848,#33531,#33532);
#28365=AXIS2_PLACEMENT_3D('',#52849,#33533,#33534);
#28366=AXIS2_PLACEMENT_3D('',#52851,#33535,#33536);
#28367=AXIS2_PLACEMENT_3D('',#52853,#33538,#33539);
#28368=AXIS2_PLACEMENT_3D('',#52856,#33541,#33542);
#28369=AXIS2_PLACEMENT_3D('',#52857,#33543,#33544);
#28370=AXIS2_PLACEMENT_3D('',#52859,#33545,#33546);
#28371=AXIS2_PLACEMENT_3D('',#52861,#33548,#33549);
#28372=AXIS2_PLACEMENT_3D('',#52864,#33551,#33552);
#28373=AXIS2_PLACEMENT_3D('',#52865,#33553,#33554);
#28374=AXIS2_PLACEMENT_3D('',#52867,#33555,#33556);
#28375=AXIS2_PLACEMENT_3D('',#52869,#33558,#33559);
#28376=AXIS2_PLACEMENT_3D('',#52872,#33561,#33562);
#28377=AXIS2_PLACEMENT_3D('',#52873,#33563,#33564);
#28378=AXIS2_PLACEMENT_3D('',#52879,#33568,#33569);
#28379=AXIS2_PLACEMENT_3D('',#52883,#33572,#33573);
#28380=AXIS2_PLACEMENT_3D('',#52887,#33576,#33577);
#28381=AXIS2_PLACEMENT_3D('',#52891,#33580,#33581);
#28382=AXIS2_PLACEMENT_3D('',#52895,#33584,#33585);
#28383=AXIS2_PLACEMENT_3D('',#52897,#33587,#33588);
#28384=AXIS2_PLACEMENT_3D('',#52903,#33592,#33593);
#28385=AXIS2_PLACEMENT_3D('',#52907,#33596,#33597);
#28386=AXIS2_PLACEMENT_3D('',#52911,#33600,#33601);
#28387=AXIS2_PLACEMENT_3D('',#52915,#33604,#33605);
#28388=AXIS2_PLACEMENT_3D('',#52919,#33608,#33609);
#28389=AXIS2_PLACEMENT_3D('',#52921,#33611,#33612);
#28390=AXIS2_PLACEMENT_3D('',#52927,#33616,#33617);
#28391=AXIS2_PLACEMENT_3D('',#52931,#33620,#33621);
#28392=AXIS2_PLACEMENT_3D('',#52935,#33624,#33625);
#28393=AXIS2_PLACEMENT_3D('',#52939,#33628,#33629);
#28394=AXIS2_PLACEMENT_3D('',#52943,#33632,#33633);
#28395=AXIS2_PLACEMENT_3D('',#52947,#33636,#33637);
#28396=AXIS2_PLACEMENT_3D('',#52951,#33640,#33641);
#28397=AXIS2_PLACEMENT_3D('',#52953,#33643,#33644);
#28398=AXIS2_PLACEMENT_3D('',#52959,#33648,#33649);
#28399=AXIS2_PLACEMENT_3D('',#52963,#33652,#33653);
#28400=AXIS2_PLACEMENT_3D('',#52967,#33656,#33657);
#28401=AXIS2_PLACEMENT_3D('',#52971,#33660,#33661);
#28402=AXIS2_PLACEMENT_3D('',#52975,#33664,#33665);
#28403=AXIS2_PLACEMENT_3D('',#52979,#33668,#33669);
#28404=AXIS2_PLACEMENT_3D('',#52983,#33672,#33673);
#28405=AXIS2_PLACEMENT_3D('',#52985,#33675,#33676);
#33443=DIRECTION('axis',(0.,0.,1.));
#33444=DIRECTION('refdir',(1.,0.,0.));
#33445=DIRECTION('center_axis',(1.,0.,0.));
#33446=DIRECTION('ref_axis',(0.,0.,-1.));
#33447=DIRECTION('center_axis',(-1.,0.,0.));
#33448=DIRECTION('ref_axis',(0.,0.,-1.));
#33449=DIRECTION('',(0.707106781186548,-8.65956056235493E-17,0.707106781186547));
#33450=DIRECTION('center_axis',(1.,0.,0.));
#33451=DIRECTION('ref_axis',(0.,0.,-1.));
#33452=DIRECTION('center_axis',(1.,0.,0.));
#33453=DIRECTION('ref_axis',(0.,0.,-1.));
#33454=DIRECTION('',(0.,-1.,0.));
#33455=DIRECTION('',(0.,0.,1.));
#33456=DIRECTION('',(0.,1.,0.));
#33457=DIRECTION('',(0.,0.,1.));
#33458=DIRECTION('',(0.,-1.,0.));
#33459=DIRECTION('',(0.,0.,-1.));
#33460=DIRECTION('',(0.,1.,0.));
#33461=DIRECTION('',(0.,0.,1.));
#33462=DIRECTION('center_axis',(1.,0.,0.));
#33463=DIRECTION('ref_axis',(0.,0.,-1.));
#33464=DIRECTION('center_axis',(1.,0.,0.));
#33465=DIRECTION('ref_axis',(0.,0.,-1.));
#33466=DIRECTION('center_axis',(1.,0.,0.));
#33467=DIRECTION('ref_axis',(0.,0.,-1.));
#33468=DIRECTION('center_axis',(1.,0.,0.));
#33469=DIRECTION('ref_axis',(0.,0.,-1.));
#33470=DIRECTION('',(0.,-1.,0.));
#33471=DIRECTION('',(0.,0.,1.));
#33472=DIRECTION('',(0.,1.,0.));
#33473=DIRECTION('',(0.,0.,-1.));
#33474=DIRECTION('',(0.,-1.,0.));
#33475=DIRECTION('',(0.,0.,-1.));
#33476=DIRECTION('',(0.,0.,-1.));
#33477=DIRECTION('',(0.,1.,0.));
#33478=DIRECTION('',(0.,0.,-1.));
#33479=DIRECTION('',(0.,-1.,0.));
#33480=DIRECTION('',(0.,0.,1.));
#33481=DIRECTION('',(0.,1.,0.));
#33482=DIRECTION('center_axis',(1.,0.,0.));
#33483=DIRECTION('ref_axis',(0.,0.,-1.));
#33484=DIRECTION('center_axis',(1.,0.,0.));
#33485=DIRECTION('ref_axis',(0.,0.,-1.));
#33486=DIRECTION('center_axis',(1.,0.,0.));
#33487=DIRECTION('ref_axis',(0.,0.,-1.));
#33488=DIRECTION('center_axis',(-1.,0.,0.));
#33489=DIRECTION('ref_axis',(0.,0.,-1.));
#33490=DIRECTION('',(-1.,0.,0.));
#33491=DIRECTION('center_axis',(1.,0.,0.));
#33492=DIRECTION('ref_axis',(0.,0.,-1.));
#33493=DIRECTION('center_axis',(1.,0.,0.));
#33494=DIRECTION('ref_axis',(0.,0.,-1.));
#33495=DIRECTION('center_axis',(-1.,0.,0.));
#33496=DIRECTION('ref_axis',(0.,0.,-1.));
#33497=DIRECTION('',(0.707106781186548,-8.65956056235493E-17,0.707106781186547));
#33498=DIRECTION('center_axis',(-1.,0.,0.));
#33499=DIRECTION('ref_axis',(0.,0.,-1.));
#33500=DIRECTION('',(-1.,0.,0.));
#33501=DIRECTION('center_axis',(1.,0.,0.));
#33502=DIRECTION('ref_axis',(0.,0.,-1.));
#33503=DIRECTION('center_axis',(1.,0.,0.));
#33504=DIRECTION('ref_axis',(0.,0.,-1.));
#33505=DIRECTION('center_axis',(-1.,0.,0.));
#33506=DIRECTION('ref_axis',(0.,0.,-1.));
#33507=DIRECTION('',(0.707106781186548,-8.65956056235493E-17,0.707106781186547));
#33508=DIRECTION('center_axis',(-1.,0.,0.));
#33509=DIRECTION('ref_axis',(0.,0.,-1.));
#33510=DIRECTION('',(-1.,0.,0.));
#33511=DIRECTION('center_axis',(1.,0.,0.));
#33512=DIRECTION('ref_axis',(0.,0.,-1.));
#33513=DIRECTION('center_axis',(1.,0.,0.));
#33514=DIRECTION('ref_axis',(0.,0.,-1.));
#33515=DIRECTION('center_axis',(-1.,0.,0.));
#33516=DIRECTION('ref_axis',(0.,0.,-1.));
#33517=DIRECTION('',(0.707106781186548,-8.65956056235493E-17,0.707106781186547));
#33518=DIRECTION('center_axis',(-1.,0.,0.));
#33519=DIRECTION('ref_axis',(0.,0.,-1.));
#33520=DIRECTION('',(-1.,0.,0.));
#33521=DIRECTION('center_axis',(1.,0.,0.));
#33522=DIRECTION('ref_axis',(0.,0.,-1.));
#33523=DIRECTION('center_axis',(1.,0.,0.));
#33524=DIRECTION('ref_axis',(0.,0.,-1.));
#33525=DIRECTION('center_axis',(-1.,0.,0.));
#33526=DIRECTION('ref_axis',(0.,0.,-1.));
#33527=DIRECTION('',(0.707106781186548,-8.65956056235493E-17,0.707106781186547));
#33528=DIRECTION('center_axis',(-1.,0.,0.));
#33529=DIRECTION('ref_axis',(0.,0.,-1.));
#33530=DIRECTION('',(-1.,0.,0.));
#33531=DIRECTION('center_axis',(1.,0.,0.));
#33532=DIRECTION('ref_axis',(0.,0.,-1.));
#33533=DIRECTION('center_axis',(1.,0.,0.));
#33534=DIRECTION('ref_axis',(0.,0.,-1.));
#33535=DIRECTION('center_axis',(-1.,0.,0.));
#33536=DIRECTION('ref_axis',(0.,0.,-1.));
#33537=DIRECTION('',(0.707106781186548,-8.65956056235493E-17,0.707106781186547));
#33538=DIRECTION('center_axis',(-1.,0.,0.));
#33539=DIRECTION('ref_axis',(0.,0.,-1.));
#33540=DIRECTION('',(-1.,0.,0.));
#33541=DIRECTION('center_axis',(1.,0.,0.));
#33542=DIRECTION('ref_axis',(0.,0.,-1.));
#33543=DIRECTION('center_axis',(1.,0.,0.));
#33544=DIRECTION('ref_axis',(0.,0.,-1.));
#33545=DIRECTION('center_axis',(-1.,0.,0.));
#33546=DIRECTION('ref_axis',(0.,0.,-1.));
#33547=DIRECTION('',(0.707106781186548,-8.65956056235493E-17,0.707106781186547));
#33548=DIRECTION('center_axis',(-1.,0.,0.));
#33549=DIRECTION('ref_axis',(0.,0.,-1.));
#33550=DIRECTION('',(-1.,0.,0.));
#33551=DIRECTION('center_axis',(1.,0.,0.));
#33552=DIRECTION('ref_axis',(0.,0.,-1.));
#33553=DIRECTION('center_axis',(1.,0.,0.));
#33554=DIRECTION('ref_axis',(0.,0.,-1.));
#33555=DIRECTION('center_axis',(-1.,0.,0.));
#33556=DIRECTION('ref_axis',(0.,0.,-1.));
#33557=DIRECTION('',(0.707106781186548,-8.65956056235493E-17,0.707106781186547));
#33558=DIRECTION('center_axis',(-1.,0.,0.));
#33559=DIRECTION('ref_axis',(0.,0.,-1.));
#33560=DIRECTION('',(-1.,0.,0.));
#33561=DIRECTION('center_axis',(1.,0.,0.));
#33562=DIRECTION('ref_axis',(0.,0.,-1.));
#33563=DIRECTION('center_axis',(0.,1.,0.));
#33564=DIRECTION('ref_axis',(0.,0.,1.));
#33565=DIRECTION('',(0.,0.,1.));
#33566=DIRECTION('',(1.,0.,0.));
#33567=DIRECTION('',(1.,0.,0.));
#33568=DIRECTION('center_axis',(0.,0.,1.));
#33569=DIRECTION('ref_axis',(0.,-1.,0.));
#33570=DIRECTION('',(0.,-1.,0.));
#33571=DIRECTION('',(1.,0.,0.));
#33572=DIRECTION('center_axis',(0.,1.,0.));
#33573=DIRECTION('ref_axis',(0.,0.,1.));
#33574=DIRECTION('',(0.,0.,1.));
#33575=DIRECTION('',(1.,0.,0.));
#33576=DIRECTION('center_axis',(0.,0.,-1.));
#33577=DIRECTION('ref_axis',(0.,1.,0.));
#33578=DIRECTION('',(0.,1.,0.));
#33579=DIRECTION('',(1.,0.,0.));
#33580=DIRECTION('center_axis',(0.,-1.,0.));
#33581=DIRECTION('ref_axis',(0.,0.,-1.));
#33582=DIRECTION('',(0.,0.,-1.));
#33583=DIRECTION('',(1.,0.,0.));
#33584=DIRECTION('center_axis',(0.,0.,1.));
#33585=DIRECTION('ref_axis',(0.,-1.,0.));
#33586=DIRECTION('',(0.,-1.,0.));
#33587=DIRECTION('center_axis',(0.,0.,-1.));
#33588=DIRECTION('ref_axis',(0.,1.,0.));
#33589=DIRECTION('',(0.,1.,0.));
#33590=DIRECTION('',(1.,0.,0.));
#33591=DIRECTION('',(1.,0.,0.));
#33592=DIRECTION('center_axis',(0.,-1.,0.));
#33593=DIRECTION('ref_axis',(0.,0.,-1.));
#33594=DIRECTION('',(0.,0.,-1.));
#33595=DIRECTION('',(1.,0.,0.));
#33596=DIRECTION('center_axis',(0.,0.,1.));
#33597=DIRECTION('ref_axis',(0.,-1.,0.));
#33598=DIRECTION('',(0.,-1.,0.));
#33599=DIRECTION('',(1.,0.,0.));
#33600=DIRECTION('center_axis',(0.,1.,0.));
#33601=DIRECTION('ref_axis',(0.,0.,1.));
#33602=DIRECTION('',(0.,0.,1.));
#33603=DIRECTION('',(1.,0.,0.));
#33604=DIRECTION('center_axis',(0.,0.,-1.));
#33605=DIRECTION('ref_axis',(0.,1.,0.));
#33606=DIRECTION('',(0.,1.,0.));
#33607=DIRECTION('',(1.,0.,0.));
#33608=DIRECTION('center_axis',(0.,1.,0.));
#33609=DIRECTION('ref_axis',(0.,0.,1.));
#33610=DIRECTION('',(0.,0.,1.));
#33611=DIRECTION('center_axis',(0.707106781186545,0.,-0.70710678118655));
#33612=DIRECTION('ref_axis',(-0.70710678118655,0.,-0.707106781186545));
#33613=DIRECTION('',(-0.577350269189627,-0.577350269189627,-0.577350269189623));
#33614=DIRECTION('',(0.,1.,0.));
#33615=DIRECTION('',(-0.577350269189627,-0.577350269189627,-0.577350269189623));
#33616=DIRECTION('center_axis',(0.707106781186548,-0.707106781186548,0.));
#33617=DIRECTION('ref_axis',(0.,0.,-1.));
#33618=DIRECTION('',(-0.577350269189629,-0.577350269189629,0.57735026918962));
#33619=DIRECTION('',(0.,0.,-1.));
#33620=DIRECTION('center_axis',(0.707106781186542,0.,0.707106781186553));
#33621=DIRECTION('ref_axis',(0.707106781186553,0.,-0.707106781186542));
#33622=DIRECTION('',(-0.577350269189629,0.577350269189629,0.57735026918962));
#33623=DIRECTION('',(0.,-1.,0.));
#33624=DIRECTION('center_axis',(0.707106781186548,0.707106781186548,0.));
#33625=DIRECTION('ref_axis',(0.,0.,-1.));
#33626=DIRECTION('',(-0.577350269189629,0.577350269189629,-0.57735026918962));
#33627=DIRECTION('',(0.,0.,1.));
#33628=DIRECTION('center_axis',(0.707106781186542,0.,-0.707106781186553));
#33629=DIRECTION('ref_axis',(-0.707106781186553,0.,-0.707106781186542));
#33630=DIRECTION('',(-0.577350269189629,-0.577350269189629,-0.57735026918962));
#33631=DIRECTION('',(0.,1.,0.));
#33632=DIRECTION('center_axis',(0.707106781186548,-0.707106781186548,0.));
#33633=DIRECTION('ref_axis',(0.,0.,-1.));
#33634=DIRECTION('',(0.,0.,-1.));
#33635=DIRECTION('',(-0.577350269189627,-0.577350269189627,0.577350269189623));
#33636=DIRECTION('center_axis',(0.707106781186545,0.,0.70710678118655));
#33637=DIRECTION('ref_axis',(0.70710678118655,0.,-0.707106781186545));
#33638=DIRECTION('',(0.,-1.,0.));
#33639=DIRECTION('',(-0.577350269189626,-0.577350269189626,0.577350269189626));
#33640=DIRECTION('center_axis',(0.707106781186548,-0.707106781186548,0.));
#33641=DIRECTION('ref_axis',(0.,0.,-1.));
#33642=DIRECTION('',(0.,0.,-1.));
#33643=DIRECTION('center_axis',(0.,-1.,0.));
#33644=DIRECTION('ref_axis',(0.,0.,-1.));
#33645=DIRECTION('',(1.,0.,0.));
#33646=DIRECTION('',(0.,0.,1.));
#33647=DIRECTION('',(1.,0.,0.));
#33648=DIRECTION('center_axis',(0.,0.,1.));
#33649=DIRECTION('ref_axis',(0.,-1.,0.));
#33650=DIRECTION('',(1.,0.,0.));
#33651=DIRECTION('',(0.,1.,0.));
#33652=DIRECTION('center_axis',(0.,-1.,0.));
#33653=DIRECTION('ref_axis',(0.,0.,-1.));
#33654=DIRECTION('',(1.,0.,0.));
#33655=DIRECTION('',(0.,0.,1.));
#33656=DIRECTION('center_axis',(0.,0.,-1.));
#33657=DIRECTION('ref_axis',(0.,1.,0.));
#33658=DIRECTION('',(1.,0.,0.));
#33659=DIRECTION('',(0.,-1.,0.));
#33660=DIRECTION('center_axis',(0.,0.,-1.));
#33661=DIRECTION('ref_axis',(0.,1.,0.));
#33662=DIRECTION('',(0.,-1.,0.));
#33663=DIRECTION('',(1.,0.,0.));
#33664=DIRECTION('center_axis',(0.,-1.,0.));
#33665=DIRECTION('ref_axis',(0.,0.,-1.));
#33666=DIRECTION('',(1.,0.,0.));
#33667=DIRECTION('',(0.,0.,1.));
#33668=DIRECTION('center_axis',(0.,0.,1.));
#33669=DIRECTION('ref_axis',(0.,-1.,0.));
#33670=DIRECTION('',(1.,0.,0.));
#33671=DIRECTION('',(0.,1.,0.));
#33672=DIRECTION('center_axis',(0.,1.,0.));
#33673=DIRECTION('ref_axis',(0.,0.,1.));
#33674=DIRECTION('',(0.,0.,-1.));
#33675=DIRECTION('center_axis',(1.,0.,0.));
#33676=DIRECTION('ref_axis',(0.,0.,-1.));
#52751=CARTESIAN_POINT('',(0.,0.,0.));
#52752=CARTESIAN_POINT('Origin',(19.814,44.696,24.89));
#52753=CARTESIAN_POINT('',(19.689,44.696,26.668));
#52754=CARTESIAN_POINT('Origin',(19.689,44.696,24.89));
#52755=CARTESIAN_POINT('',(19.939,44.696,26.918));
#52756=CARTESIAN_POINT('',(19.814,44.696,26.793));
#52757=CARTESIAN_POINT('Origin',(19.939,44.696,24.89));
#52758=CARTESIAN_POINT('Origin',(19.939,58.158,0.));
#52759=CARTESIAN_POINT('',(19.939,50.584,14.4732));
#52760=CARTESIAN_POINT('',(19.939,41.694,14.4732));
#52761=CARTESIAN_POINT('',(19.939,49.776,14.4732));
#52762=CARTESIAN_POINT('',(19.939,50.584,-14.4732));
#52763=CARTESIAN_POINT('',(19.939,50.584,7.0866));
#52764=CARTESIAN_POINT('',(19.939,41.694,-14.4732));
#52765=CARTESIAN_POINT('',(19.939,54.221,-14.4732));
#52766=CARTESIAN_POINT('',(19.939,41.694,-27.767));
#52767=CARTESIAN_POINT('',(19.939,41.694,-7.0866));
#52768=CARTESIAN_POINT('',(19.939,74.622,-27.767));
#52769=CARTESIAN_POINT('',(19.939,49.776,-27.767));
#52770=CARTESIAN_POINT('',(19.939,74.622,27.767));
#52771=CARTESIAN_POINT('',(19.939,74.622,-14.0335));
#52772=CARTESIAN_POINT('',(19.939,41.694,27.767));
#52773=CARTESIAN_POINT('',(19.939,66.54,27.767));
#52774=CARTESIAN_POINT('',(19.939,41.694,14.0335));
#52775=CARTESIAN_POINT('',(19.939,44.696,-16.262));
#52776=CARTESIAN_POINT('Origin',(19.939,44.696,-18.29));
#52777=CARTESIAN_POINT('',(19.939,71.6454,15.498));
#52778=CARTESIAN_POINT('Origin',(19.939,71.6454,13.47));
#52779=CARTESIAN_POINT('',(19.939,71.6454,26.918));
#52780=CARTESIAN_POINT('Origin',(19.939,71.6454,24.89));
#52781=CARTESIAN_POINT('',(19.939,44.696,20.318));
#52782=CARTESIAN_POINT('Origin',(19.939,44.696,18.29));
#52783=CARTESIAN_POINT('',(19.939,57.565,5.1));
#52784=CARTESIAN_POINT('',(19.939,54.26,5.1));
#52785=CARTESIAN_POINT('',(19.939,56.209,5.1));
#52786=CARTESIAN_POINT('',(19.939,54.26,16.892));
#52787=CARTESIAN_POINT('',(19.939,54.26,8.446));
#52788=CARTESIAN_POINT('',(19.939,63.912,16.892));
#52789=CARTESIAN_POINT('',(19.939,61.035,16.892));
#52790=CARTESIAN_POINT('',(19.939,63.912,7.24));
#52791=CARTESIAN_POINT('',(19.939,63.912,3.62));
#52792=CARTESIAN_POINT('',(19.939,57.565,7.24));
#52793=CARTESIAN_POINT('',(19.939,57.8615,7.24));
#52794=CARTESIAN_POINT('',(19.939,57.565,2.55));
#52795=CARTESIAN_POINT('',(19.939,57.565,-5.1));
#52796=CARTESIAN_POINT('',(19.939,57.565,-7.24));
#52797=CARTESIAN_POINT('',(19.939,57.565,-3.62));
#52798=CARTESIAN_POINT('',(19.939,63.912,-7.24));
#52799=CARTESIAN_POINT('',(19.939,61.035,-7.24));
#52800=CARTESIAN_POINT('',(19.939,63.912,-16.892));
#52801=CARTESIAN_POINT('',(19.939,63.912,-8.446));
#52802=CARTESIAN_POINT('',(19.939,54.26,-16.892));
#52803=CARTESIAN_POINT('',(19.939,56.209,-16.892));
#52804=CARTESIAN_POINT('',(19.939,54.26,-5.1));
#52805=CARTESIAN_POINT('',(19.939,54.26,-2.55));
#52806=CARTESIAN_POINT('',(19.939,57.8615,-5.1));
#52807=CARTESIAN_POINT('',(19.939,44.696,-22.862));
#52808=CARTESIAN_POINT('Origin',(19.939,44.696,-24.89));
#52809=CARTESIAN_POINT('',(19.939,71.6454,-11.442));
#52810=CARTESIAN_POINT('Origin',(19.939,71.6454,-13.47));
#52811=CARTESIAN_POINT('',(19.939,71.6454,-22.862));
#52812=CARTESIAN_POINT('Origin',(19.939,71.6454,-24.89));
#52813=CARTESIAN_POINT('Origin',(19.939,44.696,24.89));
#52814=CARTESIAN_POINT('',(16.764,44.696,26.668));
#52815=CARTESIAN_POINT('',(19.939,44.696,26.668));
#52816=CARTESIAN_POINT('Origin',(16.764,44.696,24.89));
#52817=CARTESIAN_POINT('Origin',(19.814,44.696,-18.29));
#52818=CARTESIAN_POINT('',(19.689,44.696,-16.512));
#52819=CARTESIAN_POINT('Origin',(19.689,44.696,-18.29));
#52820=CARTESIAN_POINT('',(19.814,44.696,-16.387));
#52821=CARTESIAN_POINT('Origin',(19.939,44.696,-18.29));
#52822=CARTESIAN_POINT('',(16.764,44.696,-16.512));
#52823=CARTESIAN_POINT('',(19.939,44.696,-16.512));
#52824=CARTESIAN_POINT('Origin',(16.764,44.696,-18.29));
#52825=CARTESIAN_POINT('Origin',(19.814,71.6454,-24.89));
#52826=CARTESIAN_POINT('',(19.689,71.6454,-23.112));
#52827=CARTESIAN_POINT('Origin',(19.689,71.6454,-24.89));
#52828=CARTESIAN_POINT('',(19.814,71.6454,-22.987));
#52829=CARTESIAN_POINT('Origin',(19.939,71.6454,-24.89));
#52830=CARTESIAN_POINT('',(16.764,71.6454,-23.112));
#52831=CARTESIAN_POINT('',(19.939,71.6454,-23.112));
#52832=CARTESIAN_POINT('Origin',(16.764,71.6454,-24.89));
#52833=CARTESIAN_POINT('Origin',(19.814,71.6454,13.47));
#52834=CARTESIAN_POINT('',(19.689,71.6454,15.248));
#52835=CARTESIAN_POINT('Origin',(19.689,71.6454,13.47));
#52836=CARTESIAN_POINT('',(19.814,71.6454,15.373));
#52837=CARTESIAN_POINT('Origin',(19.939,71.6454,13.47));
#52838=CARTESIAN_POINT('',(16.764,71.6454,15.248));
#52839=CARTESIAN_POINT('',(19.939,71.6454,15.248));
#52840=CARTESIAN_POINT('Origin',(16.764,71.6454,13.47));
#52841=CARTESIAN_POINT('Origin',(19.814,71.6454,-13.47));
#52842=CARTESIAN_POINT('',(19.689,71.6454,-11.692));
#52843=CARTESIAN_POINT('Origin',(19.689,71.6454,-13.47));
#52844=CARTESIAN_POINT('',(19.814,71.6454,-11.567));
#52845=CARTESIAN_POINT('Origin',(19.939,71.6454,-13.47));
#52846=CARTESIAN_POINT('',(16.764,71.6454,-11.692));
#52847=CARTESIAN_POINT('',(19.939,71.6454,-11.692));
#52848=CARTESIAN_POINT('Origin',(16.764,71.6454,-13.47));
#52849=CARTESIAN_POINT('Origin',(19.814,71.6454,24.89));
#52850=CARTESIAN_POINT('',(19.689,71.6454,26.668));
#52851=CARTESIAN_POINT('Origin',(19.689,71.6454,24.89));
#52852=CARTESIAN_POINT('',(19.814,71.6454,26.793));
#52853=CARTESIAN_POINT('Origin',(19.939,71.6454,24.89));
#52854=CARTESIAN_POINT('',(16.764,71.6454,26.668));
#52855=CARTESIAN_POINT('',(19.939,71.6454,26.668));
#52856=CARTESIAN_POINT('Origin',(16.764,71.6454,24.89));
#52857=CARTESIAN_POINT('Origin',(19.814,44.696,-24.89));
#52858=CARTESIAN_POINT('',(19.689,44.696,-23.112));
#52859=CARTESIAN_POINT('Origin',(19.689,44.696,-24.89));
#52860=CARTESIAN_POINT('',(19.814,44.696,-22.987));
#52861=CARTESIAN_POINT('Origin',(19.939,44.696,-24.89));
#52862=CARTESIAN_POINT('',(16.764,44.696,-23.112));
#52863=CARTESIAN_POINT('',(19.939,44.696,-23.112));
#52864=CARTESIAN_POINT('Origin',(16.764,44.696,-24.89));
#52865=CARTESIAN_POINT('Origin',(19.814,44.696,18.29));
#52866=CARTESIAN_POINT('',(19.689,44.696,20.068));
#52867=CARTESIAN_POINT('Origin',(19.689,44.696,18.29));
#52868=CARTESIAN_POINT('',(19.814,44.696,20.193));
#52869=CARTESIAN_POINT('Origin',(19.939,44.696,18.29));
#52870=CARTESIAN_POINT('',(16.764,44.696,20.068));
#52871=CARTESIAN_POINT('',(19.939,44.696,20.068));
#52872=CARTESIAN_POINT('Origin',(16.764,44.696,18.29));
#52873=CARTESIAN_POINT('Origin',(16.764,57.565,-7.24));
#52874=CARTESIAN_POINT('',(16.764,57.565,-7.24));
#52875=CARTESIAN_POINT('',(16.764,57.565,-5.1));
#52876=CARTESIAN_POINT('',(16.764,57.565,-3.62));
#52877=CARTESIAN_POINT('',(16.764,57.565,-7.24));
#52878=CARTESIAN_POINT('',(16.764,57.565,-5.1));
#52879=CARTESIAN_POINT('Origin',(16.764,63.912,-7.24));
#52880=CARTESIAN_POINT('',(16.764,63.912,-7.24));
#52881=CARTESIAN_POINT('',(16.764,61.035,-7.24));
#52882=CARTESIAN_POINT('',(16.764,63.912,-7.24));
#52883=CARTESIAN_POINT('Origin',(16.764,63.912,-16.892));
#52884=CARTESIAN_POINT('',(16.764,63.912,-16.892));
#52885=CARTESIAN_POINT('',(16.764,63.912,-8.446));
#52886=CARTESIAN_POINT('',(16.764,63.912,-16.892));
#52887=CARTESIAN_POINT('Origin',(16.764,54.26,-16.892));
#52888=CARTESIAN_POINT('',(16.764,54.26,-16.892));
#52889=CARTESIAN_POINT('',(16.764,56.209,-16.892));
#52890=CARTESIAN_POINT('',(16.764,54.26,-16.892));
#52891=CARTESIAN_POINT('Origin',(16.764,54.26,-5.1));
#52892=CARTESIAN_POINT('',(16.764,54.26,-5.1));
#52893=CARTESIAN_POINT('',(16.764,54.26,-2.55));
#52894=CARTESIAN_POINT('',(16.764,54.26,-5.1));
#52895=CARTESIAN_POINT('Origin',(16.764,57.565,-5.1));
#52896=CARTESIAN_POINT('',(16.764,57.8615,-5.1));
#52897=CARTESIAN_POINT('Origin',(16.764,54.26,5.1));
#52898=CARTESIAN_POINT('',(16.764,54.26,5.1));
#52899=CARTESIAN_POINT('',(16.764,57.565,5.1));
#52900=CARTESIAN_POINT('',(16.764,56.209,5.1));
#52901=CARTESIAN_POINT('',(16.764,54.26,5.1));
#52902=CARTESIAN_POINT('',(16.764,57.565,5.1));
#52903=CARTESIAN_POINT('Origin',(16.764,54.26,16.892));
#52904=CARTESIAN_POINT('',(16.764,54.26,16.892));
#52905=CARTESIAN_POINT('',(16.764,54.26,8.446));
#52906=CARTESIAN_POINT('',(16.764,54.26,16.892));
#52907=CARTESIAN_POINT('Origin',(16.764,63.912,16.892));
#52908=CARTESIAN_POINT('',(16.764,63.912,16.892));
#52909=CARTESIAN_POINT('',(16.764,61.035,16.892));
#52910=CARTESIAN_POINT('',(16.764,63.912,16.892));
#52911=CARTESIAN_POINT('Origin',(16.764,63.912,7.24));
#52912=CARTESIAN_POINT('',(16.764,63.912,7.24));
#52913=CARTESIAN_POINT('',(16.764,63.912,3.62));
#52914=CARTESIAN_POINT('',(16.764,63.912,7.24));
#52915=CARTESIAN_POINT('Origin',(16.764,57.565,7.24));
#52916=CARTESIAN_POINT('',(16.764,57.565,7.24));
#52917=CARTESIAN_POINT('',(16.764,57.8615,7.24));
#52918=CARTESIAN_POINT('',(16.764,57.565,7.24));
#52919=CARTESIAN_POINT('Origin',(16.764,57.565,5.1));
#52920=CARTESIAN_POINT('',(16.764,57.565,2.55));
#52921=CARTESIAN_POINT('Origin',(19.789,49.776,14.3232));
#52922=CARTESIAN_POINT('',(19.639,41.394,14.1732));
#52923=CARTESIAN_POINT('',(19.939,41.694,14.4732));
#52924=CARTESIAN_POINT('',(19.639,50.284,14.1732));
#52925=CARTESIAN_POINT('',(19.639,49.776,14.1732));
#52926=CARTESIAN_POINT('',(19.939,50.584,14.4732));
#52927=CARTESIAN_POINT('Origin',(19.789,41.544,14.0335));
#52928=CARTESIAN_POINT('',(19.639,41.394,28.067));
#52929=CARTESIAN_POINT('',(19.939,41.694,27.767));
#52930=CARTESIAN_POINT('',(19.639,41.394,14.0335));
#52931=CARTESIAN_POINT('Origin',(19.789,66.54,27.917));
#52932=CARTESIAN_POINT('',(19.639,74.922,28.067));
#52933=CARTESIAN_POINT('',(19.939,74.622,27.767));
#52934=CARTESIAN_POINT('',(19.639,66.54,28.067));
#52935=CARTESIAN_POINT('Origin',(19.789,74.772,-14.0335));
#52936=CARTESIAN_POINT('',(19.639,74.922,-28.067));
#52937=CARTESIAN_POINT('',(19.939,74.622,-27.767));
#52938=CARTESIAN_POINT('',(19.639,74.922,-14.0335));
#52939=CARTESIAN_POINT('Origin',(19.789,49.776,-27.917));
#52940=CARTESIAN_POINT('',(19.639,41.394,-28.067));
#52941=CARTESIAN_POINT('',(19.939,41.694,-27.767));
#52942=CARTESIAN_POINT('',(19.639,49.776,-28.067));
#52943=CARTESIAN_POINT('Origin',(19.789,41.544,-7.0866));
#52944=CARTESIAN_POINT('',(19.639,41.394,-14.1732));
#52945=CARTESIAN_POINT('',(19.639,41.394,-7.0866));
#52946=CARTESIAN_POINT('',(19.939,41.694,-14.4732));
#52947=CARTESIAN_POINT('Origin',(19.789,54.221,-14.3232));
#52948=CARTESIAN_POINT('',(19.639,50.284,-14.1732));
#52949=CARTESIAN_POINT('',(19.639,54.221,-14.1732));
#52950=CARTESIAN_POINT('',(19.939,50.584,-14.4732));
#52951=CARTESIAN_POINT('Origin',(19.789,50.434,7.0866));
#52952=CARTESIAN_POINT('',(19.639,50.284,7.0866));
#52953=CARTESIAN_POINT('Origin',(16.764,41.394,-14.1732));
#52954=CARTESIAN_POINT('',(16.764,41.394,-14.1732));
#52955=CARTESIAN_POINT('',(16.764,41.394,-14.1732));
#52956=CARTESIAN_POINT('',(16.764,41.394,-28.067));
#52957=CARTESIAN_POINT('',(16.764,41.394,-28.067));
#52958=CARTESIAN_POINT('',(16.764,41.394,-28.067));
#52959=CARTESIAN_POINT('Origin',(16.764,50.284,-14.1732));
#52960=CARTESIAN_POINT('',(16.764,50.284,-14.1732));
#52961=CARTESIAN_POINT('',(16.764,50.284,-14.1732));
#52962=CARTESIAN_POINT('',(16.764,41.394,-14.1732));
#52963=CARTESIAN_POINT('Origin',(16.764,50.284,14.1732));
#52964=CARTESIAN_POINT('',(16.764,50.284,14.1732));
#52965=CARTESIAN_POINT('',(16.764,50.284,14.1732));
#52966=CARTESIAN_POINT('',(16.764,50.284,-14.1732));
#52967=CARTESIAN_POINT('Origin',(16.764,41.394,14.1732));
#52968=CARTESIAN_POINT('',(16.764,41.394,14.1732));
#52969=CARTESIAN_POINT('',(16.764,41.394,14.1732));
#52970=CARTESIAN_POINT('',(16.764,50.284,14.1732));
#52971=CARTESIAN_POINT('Origin',(16.764,41.394,-28.067));
#52972=CARTESIAN_POINT('',(16.764,74.922,-28.067));
#52973=CARTESIAN_POINT('',(16.764,74.922,-28.067));
#52974=CARTESIAN_POINT('',(16.764,74.922,-28.067));
#52975=CARTESIAN_POINT('Origin',(16.764,41.394,28.067));
#52976=CARTESIAN_POINT('',(16.764,41.394,28.067));
#52977=CARTESIAN_POINT('',(16.764,41.394,28.067));
#52978=CARTESIAN_POINT('',(16.764,41.394,14.1732));
#52979=CARTESIAN_POINT('Origin',(16.764,74.922,28.067));
#52980=CARTESIAN_POINT('',(16.764,74.922,28.067));
#52981=CARTESIAN_POINT('',(16.764,74.922,28.067));
#52982=CARTESIAN_POINT('',(16.764,41.394,28.067));
#52983=CARTESIAN_POINT('Origin',(16.764,74.922,-28.067));
#52984=CARTESIAN_POINT('',(16.764,74.922,28.067));
#52985=CARTESIAN_POINT('Origin',(16.764,58.158,0.));
#83196=UNCERTAINTY_MEASURE_WITH_UNIT(LENGTH_MEASURE(0.01),#83220,
'DISTANCE_ACCURACY_VALUE',
'Maximum model space distance between geometric entities at asserted c
onnectivities');
#83203=UNCERTAINTY_MEASURE_WITH_UNIT(LENGTH_MEASURE(0.01),#83220,
'DISTANCE_ACCURACY_VALUE',
'Maximum model space distance between geometric entities at asserted c
onnectivities');
#83212=(
GEOMETRIC_REPRESENTATION_CONTEXT(3)
GLOBAL_UNCERTAINTY_ASSIGNED_CONTEXT((#83196))
GLOBAL_UNIT_ASSIGNED_CONTEXT((#83220,#83222,#83223))
REPRESENTATION_CONTEXT('','3D')
);
#83219=(
GEOMETRIC_REPRESENTATION_CONTEXT(3)
GLOBAL_UNCERTAINTY_ASSIGNED_CONTEXT((#83203))
GLOBAL_UNIT_ASSIGNED_CONTEXT((#83220,#83222,#83223))
REPRESENTATION_CONTEXT('','3D')
);
#83220=(
LENGTH_UNIT()
NAMED_UNIT(*)
SI_UNIT(.MILLI.,.METRE.)
);
#83222=(
NAMED_UNIT(*)
PLANE_ANGLE_UNIT()
SI_UNIT($,.RADIAN.)
);
#83223=(
NAMED_UNIT(*)
SI_UNIT($,.STERADIAN.)
SOLID_ANGLE_UNIT()
);
#83232=SHAPE_DEFINITION_REPRESENTATION(#83247,#83307);
#83247=PRODUCT_DEFINITION_SHAPE('',$,#83323);
#83307=SHAPE_REPRESENTATION('',(#28335),#83212);
#83314=PRODUCT_DEFINITION_CONTEXT('part definition',#83361,'design');
#83323=PRODUCT_DEFINITION('Beam Bracket W Acetal',
'Beam Bracket W Acetal',#83338,#83314);
#83338=PRODUCT_DEFINITION_FORMATION('',$,#83371);
#83361=APPLICATION_CONTEXT(
'Core Data for Automotive Mechanical Design Process');
#83362=PRODUCT_CONTEXT('part definition',#83361,'mechanical');
#83371=PRODUCT('Beam Bracket W Acetal','Beam Bracket W Acetal',$,(#83362));
#83386=PRESENTATION_STYLE_ASSIGNMENT((#83401));
#83401=SURFACE_STYLE_USAGE(.BOTH.,#83416);
#83416=SURFACE_SIDE_STYLE('',(#83431));
#83431=SURFACE_STYLE_FILL_AREA(#83446);
#83446=FILL_AREA_STYLE('Opaque(200,204,210)',(#83461));
#83461=FILL_AREA_STYLE_COLOUR('Opaque(200,204,210)',#83476);
#83476=COLOUR_RGB('Opaque(200,204,210)', 0.31764706, 0.68627451, 0.89019608);
ENDSEC;
END-ISO-10303-21;
